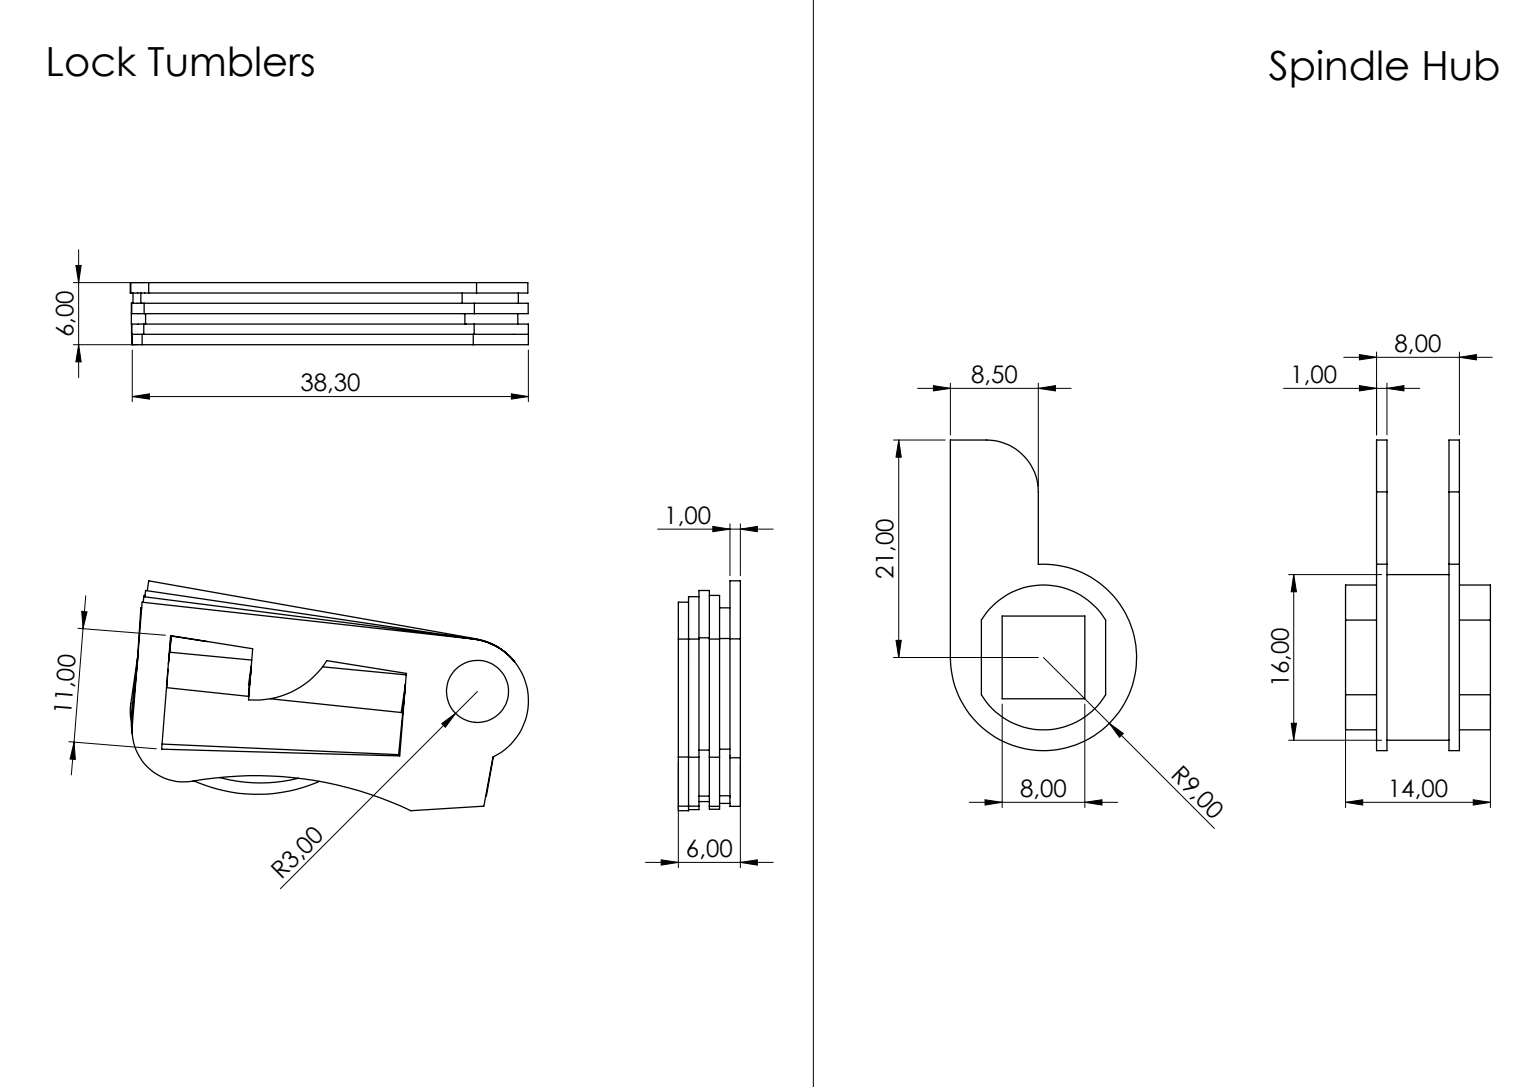
ISO-10303-21;
HEADER;
FILE_DESCRIPTION (('STEP AP214'),
    '1' );
FILE_NAME ('Spindle Hub.step',
    '2026-10-06T13:23:30',
    ( '' ),
    ( '' ),
    'SwSTEP 2.0',
    'SolidWorks 2020',
    '' );
FILE_SCHEMA (( 'AUTOMOTIVE_DESIGN' ));
ENDSEC;

DATA;
#2=FACE_OUTER_BOUND ( 'NONE', #19323, .T. ) ;
#35=FACE_OUTER_BOUND ( 'NONE', #21489, .T. ) ;
#39=ORIENTED_EDGE ( 'NONE', *, *, #18140, .F. ) ;
#55=ORIENTED_EDGE ( 'NONE', *, *, #18140, .T. ) ;
#134=LINE ( 'NONE', #14635, #4183 ) ;
#182=UNCERTAINTY_MEASURE_WITH_UNIT (LENGTH_MEASURE( 1.000000000000000082E-05 ), #19737, 'distance_accuracy_value', 'NONE');
#193=ORIENTED_EDGE ( 'NONE', *, *, #5602, .T. ) ;
#231=EDGE_CURVE ( 'NONE', #11233, #3677, #3985, .T. ) ;
#251=CARTESIAN_POINT ( 'NONE',  ( 10.50000000010000001, 20.50000000000000000, -150.5552959529999839 ) ) ;
#291=CARTESIAN_POINT ( 'NONE',  ( -0.7499999998410000757, 41.50000000000000000, -139.5552959529999839 ) ) ;
#295=ORIENTED_EDGE ( 'NONE', *, *, #21236, .T. ) ;
#312=DIRECTION ( 'NONE',  ( 2.257144641399999941E-12, -4.009147065140000298E-51, 1.000000000000000000 ) ) ;
#362=AXIS2_PLACEMENT_3D ( 'NONE', #6405, #22711, #20943 ) ;
#418=PLANE ( 'NONE',  #1885 ) ;
#426=FACE_OUTER_BOUND ( 'NONE', #14985, .T. ) ;
#436=ORIENTED_EDGE ( 'NONE', *, *, #7654, .T. ) ;
#439=ORIENTED_EDGE ( 'NONE', *, *, #4229, .F. ) ;
#486=AXIS2_PLACEMENT_3D ( 'NONE', #13907, #11751, #12111 ) ;
#542=ORIENTED_EDGE ( 'NONE', *, *, #17707, .F. ) ;
#547=DIRECTION ( 'NONE',  ( -2.257144641399999941E-12, 0.000000000000000000, -1.000000000000000000 ) ) ;
#628=CARTESIAN_POINT ( 'NONE',  ( 12.50000000010000001, 24.10555127549999810, -150.5552959529999839 ) ) ;
#665=ADVANCED_FACE ( 'NONE', ( #6439 ), #20974, .T. ) ;
#705=ORIENTED_EDGE ( 'NONE', *, *, #23377, .F. ) ;
#708=ORIENTED_EDGE ( 'NONE', *, *, #12053, .T. ) ;
#731=AXIS2_PLACEMENT_3D ( 'NONE', #8142, #11836, #22803 ) ;
#762=CARTESIAN_POINT ( 'NONE',  ( 12.50000000010000001, 20.50000000000000000, -147.5552959529999839 ) ) ;
#781=PRODUCT_DEFINITION ( 'UNKNOWN', '', #11904, #8501 ) ;
#813=CARTESIAN_POINT ( 'NONE',  ( 6.500000000149999124, 20.50000000000000000, -143.5552959529999839 ) ) ;
#855=ORIENTED_EDGE ( 'NONE', *, *, #15175, .F. ) ;
#860=ORIENTED_EDGE ( 'NONE', *, *, #19332, .F. ) ;
#899=FACE_OUTER_BOUND ( 'NONE', #6411, .T. ) ;
#901=CARTESIAN_POINT ( 'NONE',  ( 0.5000000001500000124, 16.89444872450000190, -143.5552959529999839 ) ) ;
#999=DIRECTION ( 'NONE',  ( 1.000000000000000000, 0.000000000000000000, -2.256131789327549967E-12 ) ) ;
#1028=CARTESIAN_POINT ( 'NONE',  ( 6.500000000159999125, 12.50000000000000000, -140.5552959529999839 ) ) ;
#1080=DIRECTION ( 'NONE',  ( 1.000000000000000000, -1.190078432789999897E-50, -2.257144641399999941E-12 ) ) ;
#1107=EDGE_CURVE ( 'NONE', #9556, #20751, #13681, .T. ) ;
#1109=EDGE_LOOP ( 'NONE', ( #4239, #8656, #12056, #15119 ) ) ;
#1120=DIRECTION ( 'NONE',  ( 2.257144641399999941E-12, -4.009147065140000298E-51, 1.000000000000000000 ) ) ;
#1121=VECTOR ( 'NONE', #19395, 1000.000000000000000 ) ;
#1130=ORIENTED_EDGE ( 'NONE', *, *, #23377, .T. ) ;
#1161=DIRECTION ( 'NONE',  ( 1.000000000000000000, 0.000000000000000000, 0.000000000000000000 ) ) ;
#1163=DIRECTION ( 'NONE',  ( 2.257144641399999941E-12, -4.009147065140000298E-51, 1.000000000000000000 ) ) ;
#1177=DIRECTION ( 'NONE',  ( 1.000000000000000000, 0.000000000000000000, -2.257453483404484831E-12 ) ) ;
#1188=DIRECTION ( 'NONE',  ( 1.000000000000000000, 0.000000000000000000, -2.257144641399999941E-12 ) ) ;
#1201=ORIENTED_EDGE ( 'NONE', *, *, #14324, .T. ) ;
#1232=ORIENTED_EDGE ( 'NONE', *, *, #20162, .F. ) ;
#1337=CARTESIAN_POINT ( 'NONE',  ( 1.000000000140000012, 41.50000000000000000, -147.0552959529999839 ) ) ;
#1349=CARTESIAN_POINT ( 'NONE',  ( 6.500000000140000012, 20.50000000000000000, -147.5552959529999839 ) ) ;
#1366=CARTESIAN_POINT ( 'NONE',  ( 2.500000000150000012, 24.50000000000000000, -143.5552959529999839 ) ) ;
#1369=VERTEX_POINT ( 'NONE', #15757 ) ;
#1379=EDGE_CURVE ( 'NONE', #9692, #10188, #2914, .T. ) ;
#1491=ORIENTED_EDGE ( 'NONE', *, *, #21184, .T. ) ;
#1565=CARTESIAN_POINT ( 'NONE',  ( -2.499999999859999988, 20.50000000000000000, -147.5552959529999839 ) ) ;
#1588=EDGE_CURVE ( 'NONE', #2933, #20660, #20036, .T. ) ;
#1620=CARTESIAN_POINT ( 'NONE',  ( 0.5000000001590000354, 20.50000000000000000, -139.5552959529999839 ) ) ;
#1692=ADVANCED_FACE ( 'NONE', ( #6899 ), #14167, .F. ) ;
#1695=EDGE_CURVE ( 'NONE', #8517, #8429, #19003, .T. ) ;
#1735=DIRECTION ( 'NONE',  ( 2.256861364460000137E-12, 0.000000000000000000, 1.000000000000000000 ) ) ;
#1788=CARTESIAN_POINT ( 'NONE',  ( -2.499999999839999987, 41.50000000000000000, -140.0552959529999839 ) ) ;
#1885=AXIS2_PLACEMENT_3D ( 'NONE', #17176, #2446, #9900 ) ;
#1915=CARTESIAN_POINT ( 'NONE',  ( -2.499999999839999987, 31.00000000000000000, -139.5552959529999839 ) ) ;
#1925=DIRECTION ( 'NONE',  ( 1.000000000000000000, 0.000000000000000000, -2.258609965721802837E-12 ) ) ;
#1960=CARTESIAN_POINT ( 'NONE',  ( -2.499999999859999988, 41.50000000000000000, -147.5552959529999839 ) ) ;
#2005=ORIENTED_EDGE ( 'NONE', *, *, #2166, .T. ) ;
#2013=ADVANCED_FACE ( 'NONE', ( #19771, #23333 ), #3696, .T. ) ;
#2034=DIRECTION ( 'NONE',  ( 1.000000000000000000, 0.000000000000000000, -2.257144641399999941E-12 ) ) ;
#2135=VECTOR ( 'NONE', #11700, 1000.000000000000000 ) ;
#2162=DIRECTION ( 'NONE',  ( 0.000000000000000000, -1.000000000000000000, 0.000000000000000000 ) ) ;
#2164=VERTEX_POINT ( 'NONE', #16015 ) ;
#2166=EDGE_CURVE ( 'NONE', #14118, #10634, #8177, .T. ) ;
#2167=AXIS2_PLACEMENT_3D ( 'NONE', #6419, #4646, #10091 ) ;
#2168=EDGE_LOOP ( 'NONE', ( #4075, #9774, #2218, #5035 ) ) ;
#2216=VECTOR ( 'NONE', #13785, 1000.000000000000000 ) ;
#2218=ORIENTED_EDGE ( 'NONE', *, *, #14621, .F. ) ;
#2254=ORIENTED_EDGE ( 'NONE', *, *, #12139, .F. ) ;
#2278=AXIS2_PLACEMENT_3D ( 'NONE', #12325, #19839, #14245 ) ;
#2285=DIRECTION ( 'NONE',  ( 1.000000000000000000, -1.190078432789999897E-50, -2.257144641399999941E-12 ) ) ;
#2341=ORIENTED_EDGE ( 'NONE', *, *, #15619, .F. ) ;
#2425=STYLED_ITEM ( 'NONE', ( #4984 ), #18345 ) ;
#2446=DIRECTION ( 'NONE',  ( 2.257144641399999941E-12, -4.009147065140000298E-51, 1.000000000000000000 ) ) ;
#2493=LINE ( 'NONE', #13417, #5918 ) ;
#2504=EDGE_LOOP ( 'NONE', ( #2554, #7882, #8397, #3230 ) ) ;
#2510=EDGE_LOOP ( 'NONE', ( #11261, #16222, #18656, #11978 ) ) ;
#2515=EDGE_CURVE ( 'NONE', #12071, #8946, #22656, .T. ) ;
#2531=DIRECTION ( 'NONE',  ( 2.257144641404620116E-12, 2.777754792983395132E-24, 1.000000000000000000 ) ) ;
#2538=DIRECTION ( 'NONE',  ( 0.000000000000000000, -1.000000000000000000, 0.000000000000000000 ) ) ;
#2540=ADVANCED_FACE ( 'NONE', ( #899 ), #4099, .F. ) ;
#2554=ORIENTED_EDGE ( 'NONE', *, *, #15296, .F. ) ;
#2632=DIRECTION ( 'NONE',  ( -2.257144641399999941E-12, 4.009147065140000298E-51, -1.000000000000000000 ) ) ;
#2653=APPLICATION_CONTEXT ( 'automotive_design' ) ;
#2665=CARTESIAN_POINT ( 'NONE',  ( 6.500000000170000014, 20.50000000000000000, -136.5552959530000123 ) ) ;
#2682=DIRECTION ( 'NONE',  ( 1.000000000000000000, -1.190078432789999897E-50, -2.257144641399999941E-12 ) ) ;
#2703=ORIENTED_EDGE ( 'NONE', *, *, #14053, .F. ) ;
#2716=VERTEX_POINT ( 'NONE', #23128 ) ;
#2740=FACE_OUTER_BOUND ( 'NONE', #2504, .T. ) ;
#2744=AXIS2_PLACEMENT_3D ( 'NONE', #22872, #2531, #4664 ) ;
#2748=DIRECTION ( 'NONE',  ( -2.257144641399999941E-12, 0.000000000000000000, -1.000000000000000000 ) ) ;
#2758=VERTEX_POINT ( 'NONE', #1960 ) ;
#2824=LINE ( 'NONE', #22941, #17455 ) ;
#2858=ORIENTED_EDGE ( 'NONE', *, *, #5935, .T. ) ;
#2869=DIRECTION ( 'NONE',  ( 3.882490197650000213E-51, -1.000000000000000000, -4.009147065150000317E-51 ) ) ;
#2874=AXIS2_PLACEMENT_3D ( 'NONE', #16722, #23523, #18291 ) ;
#2914=LINE ( 'NONE', #1366, #9859 ) ;
#2933=VERTEX_POINT ( 'NONE', #628 ) ;
#2954=ORIENTED_EDGE ( 'NONE', *, *, #12303, .T. ) ;
#3018=CARTESIAN_POINT ( 'NONE',  ( 2.500000000170000014, 24.50000000000000000, -136.5552959530000123 ) ) ;
#3046=DIRECTION ( 'NONE',  ( 0.000000000000000000, 1.000000000000000000, 0.000000000000000000 ) ) ;
#3063=ORIENTED_EDGE ( 'NONE', *, *, #19396, .T. ) ;
#3075=VERTEX_POINT ( 'NONE', #16916 ) ;
#3089=ORIENTED_EDGE ( 'NONE', *, *, #3888, .T. ) ;
#3121=CARTESIAN_POINT ( 'NONE',  ( 12.50000000020000002, 24.10555127549999810, -136.5552959530000123 ) ) ;
#3136=LINE ( 'NONE', #16093, #9380 ) ;
#3230=ORIENTED_EDGE ( 'NONE', *, *, #7654, .F. ) ;
#3281=DIRECTION ( 'NONE',  ( 1.000000000000000000, 0.000000000000000000, -2.256131789327550371E-12 ) ) ;
#3299=DIRECTION ( 'NONE',  ( 2.257115129720000004E-12, 0.000000000000000000, 1.000000000000000000 ) ) ;
#3387=VECTOR ( 'NONE', #12038, 1000.000000000000000 ) ;
#3463=DIRECTION ( 'NONE',  ( 2.257144641399999941E-12, -4.009147065140000298E-51, 1.000000000000000000 ) ) ;
#3481=VERTEX_POINT ( 'NONE', #18909 ) ;
#3519=VECTOR ( 'NONE', #15234, 1000.000000000000000 ) ;
#3567=DIRECTION ( 'NONE',  ( 3.882490197650000213E-51, -1.000000000000000000, -4.009147065150000317E-51 ) ) ;
#3607=ORIENTED_EDGE ( 'NONE', *, *, #10334, .T. ) ;
#3636=AXIS2_PLACEMENT_3D ( 'NONE', #5525, #11100, #23494 ) ;
#3648=DIRECTION ( 'NONE',  ( 2.257144641399999941E-12, 0.000000000000000000, 1.000000000000000000 ) ) ;
#3667=ORIENTED_EDGE ( 'NONE', *, *, #2515, .T. ) ;
#3677=VERTEX_POINT ( 'NONE', #17482 ) ;
#3678=CARTESIAN_POINT ( 'NONE',  ( 6.500000000140000012, 20.50000000000000000, -146.5552959529999839 ) ) ;
#3696=PLANE ( 'NONE',  #12169 ) ;
#3697=CARTESIAN_POINT ( 'NONE',  ( 6.500000000159999125, 20.50000000000000000, -139.5552959529999839 ) ) ;
#3745=CARTESIAN_POINT ( 'NONE',  ( 6.500000000140000012, 20.50000000000000000, -146.5552959529999839 ) ) ;
#3758=CARTESIAN_POINT ( 'NONE',  ( 6.500000000149999124, 12.50000000000000000, -143.5552959529999839 ) ) ;
#3762=CARTESIAN_POINT ( 'NONE',  ( 1.000000000160000013, 36.50000000000000000, -140.0552959529999839 ) ) ;
#3765=AXIS2_PLACEMENT_3D ( 'NONE', #11756, #1080, #2748 ) ;
#3857=VECTOR ( 'NONE', #3299, 1000.000000000000000 ) ;
#3881=VERTEX_POINT ( 'NONE', #5913 ) ;
#3888=EDGE_CURVE ( 'NONE', #8429, #10865, #16744, .T. ) ;
#3912=DIRECTION ( 'NONE',  ( 2.256988247090000272E-12, 0.000000000000000000, 1.000000000000000000 ) ) ;
#3961=LINE ( 'NONE', #1337, #23256 ) ;
#3980=ORIENTED_EDGE ( 'NONE', *, *, #17641, .F. ) ;
#3985=LINE ( 'NONE', #11218, #16794 ) ;
#4026=DIRECTION ( 'NONE',  ( 0.8571428571427679444, 0.5150787536378610421, -1.934960128632415569E-12 ) ) ;
#4075=ORIENTED_EDGE ( 'NONE', *, *, #23457, .F. ) ;
#4099=PLANE ( 'NONE',  #17649 ) ;
#4109=ADVANCED_FACE ( 'NONE', ( #6618 ), #18878, .T. ) ;
#4137=VECTOR ( 'NONE', #14049, 1000.000000000000000 ) ;
#4149=ORIENTED_EDGE ( 'NONE', *, *, #1588, .T. ) ;
#4172=CARTESIAN_POINT ( 'NONE',  ( 12.50000000010000001, 16.89444872450000190, -143.5552959529999839 ) ) ;
#4183=VECTOR ( 'NONE', #21903, 1000.000000000000000 ) ;
#4224=EDGE_CURVE ( 'NONE', #14338, #2164, #14719, .T. ) ;
#4229=EDGE_CURVE ( 'NONE', #21917, #14118, #5306, .T. ) ;
#4230=ORIENTED_EDGE ( 'NONE', *, *, #15873, .T. ) ;
#4239=ORIENTED_EDGE ( 'NONE', *, *, #12303, .F. ) ;
#4242=VECTOR ( 'NONE', #22137, 1000.000000000000000 ) ;
#4259=CARTESIAN_POINT ( 'NONE',  ( 6.500000000140000012, 12.50000000000000000, -146.5552959529999839 ) ) ;
#4288=LINE ( 'NONE', #251, #3519 ) ;
#4306=DIRECTION ( 'NONE',  ( 1.000000000000000000, 0.000000000000000000, -2.257144641399999941E-12 ) ) ;
#4387=EDGE_LOOP ( 'NONE', ( #11899, #9813, #15038, #4737, #7332 ) ) ;
#4440=FACE_OUTER_BOUND ( 'NONE', #19109, .T. ) ;
#4463=LINE ( 'NONE', #15052, #2135 ) ;
#4550=LINE ( 'NONE', #13709, #20192 ) ;
#4565=AXIS2_PLACEMENT_3D ( 'NONE', #10450, #21431, #8551 ) ;
#4590=CARTESIAN_POINT ( 'NONE',  ( 0.000000000000000000, 0.000000000000000000, 0.000000000000000000 ) ) ;
#4602=LINE ( 'NONE', #11718, #15573 ) ;
#4620=LINE ( 'NONE', #17342, #2216 ) ;
#4622=ORIENTED_EDGE ( 'NONE', *, *, #15648, .F. ) ;
#4636=PLANE ( 'NONE',  #486 ) ;
#4646=DIRECTION ( 'NONE',  ( 2.257144641399999941E-12, -4.009147065140000298E-51, 1.000000000000000000 ) ) ;
#4664=DIRECTION ( 'NONE',  ( -0.8571428571427679444, -0.5150787536378610421, 1.934960128632415569E-12 ) ) ;
#4736=FACE_OUTER_BOUND ( 'NONE', #23383, .T. ) ;
#4737=ORIENTED_EDGE ( 'NONE', *, *, #19081, .T. ) ;
#4748=ORIENTED_EDGE ( 'NONE', *, *, #5602, .F. ) ;
#4753=AXIS2_PLACEMENT_3D ( 'NONE', #17014, #2632, #9862 ) ;
#4757=EDGE_CURVE ( 'NONE', #17568, #9722, #13324, .T. ) ;
#4795=DIRECTION ( 'NONE',  ( 2.257144641404620116E-12, 2.777754792983395132E-24, 1.000000000000000000 ) ) ;
#4810=EDGE_LOOP ( 'NONE', ( #19167, #14249, #3607, #21619 ) ) ;
#4819=DIRECTION ( 'NONE',  ( 0.000000000000000000, -1.000000000000000000, 0.000000000000000000 ) ) ;
#4872=AXIS2_PLACEMENT_3D ( 'NONE', #5169, #12870, #23150 ) ;
#4891=ADVANCED_FACE ( 'NONE', ( #21067 ), #12002, .T. ) ;
#4950=EDGE_CURVE ( 'NONE', #10763, #5071, #22748, .T. ) ;
#4964=VECTOR ( 'NONE', #8838, 1000.000000000000000 ) ;
#4974=CARTESIAN_POINT ( 'NONE',  ( 0.5000000001340000333, 24.10555127549999810, -150.5552959529999839 ) ) ;
#4984=PRESENTATION_STYLE_ASSIGNMENT (( #19966 ) ) ;
#5010=EDGE_CURVE ( 'NONE', #3075, #8221, #18193, .T. ) ;
#5025=AXIS2_PLACEMENT_3D ( 'NONE', #4590, #17084, #1161 ) ;
#5032=EDGE_CURVE ( 'NONE', #17345, #12862, #21419, .T. ) ;
#5035=ORIENTED_EDGE ( 'NONE', *, *, #13018, .F. ) ;
#5062=LINE ( 'NONE', #12306, #11250 ) ;
#5070=CARTESIAN_POINT ( 'NONE',  ( 6.500000000159999125, 20.50000000000000000, -139.5552959529999839 ) ) ;
#5071=VERTEX_POINT ( 'NONE', #4259 ) ;
#5111=CARTESIAN_POINT ( 'NONE',  ( 0.5000000001659999915, 16.89444872450000190, -136.5552959530000123 ) ) ;
#5169=CARTESIAN_POINT ( 'NONE',  ( 6.500000000140000012, 20.50000000000000000, -147.5552959529999839 ) ) ;
#5170=AXIS2_PLACEMENT_3D ( 'NONE', #1349, #1120, #15847 ) ;
#5179=ADVANCED_FACE ( 'NONE', ( #5917 ), #18423, .T. ) ;
#5210=CARTESIAN_POINT ( 'NONE',  ( -0.7499999998590000105, 41.50000000000000000, -147.5552959529999839 ) ) ;
#5222=DIRECTION ( 'NONE',  ( 0.000000000000000000, 4.009147065150000317E-51, -1.000000000000000000 ) ) ;
#5257=ORIENTED_EDGE ( 'NONE', *, *, #16090, .T. ) ;
#5282=FACE_OUTER_BOUND ( 'NONE', #2510, .T. ) ;
#5306=LINE ( 'NONE', #14239, #17777 ) ;
#5338=AXIS2_PLACEMENT_3D ( 'NONE', #901, #2682, #8371 ) ;
#5369=AXIS2_PLACEMENT_3D ( 'NONE', #6275, #13783, #17460 ) ;
#5474=EDGE_LOOP ( 'NONE', ( #21908, #2254, #20686, #10327, #9134 ) ) ;
#5496=CARTESIAN_POINT ( 'NONE',  ( 6.500000000149999124, 20.50000000000000000, -143.5552959529999839 ) ) ;
#5525=CARTESIAN_POINT ( 'NONE',  ( 1.000000000140000012, 36.50000000000000000, -147.5552959529999839 ) ) ;
#5548=CYLINDRICAL_SURFACE ( 'NONE', #2874, 7.000000000000000888 ) ;
#5579=FACE_BOUND ( 'NONE', #14822, .T. ) ;
#5584=CARTESIAN_POINT ( 'NONE',  ( 6.000000000140000012, 29.48610037779999971, -147.5552959529999839 ) ) ;
#5602=EDGE_CURVE ( 'NONE', #21645, #9539, #17282, .T. ) ;
#5649=VECTOR ( 'NONE', #2162, 1000.000000000000000 ) ;
#5694=FACE_OUTER_BOUND ( 'NONE', #5474, .T. ) ;
#5731=FACE_BOUND ( 'NONE', #2168, .T. ) ;
#5901=EDGE_LOOP ( 'NONE', ( #14706, #6579, #1130, #193 ) ) ;
#5913=CARTESIAN_POINT ( 'NONE',  ( 0.5000000001409999895, 24.10555127549999810, -147.5552959529999839 ) ) ;
#5917=FACE_OUTER_BOUND ( 'NONE', #10664, .T. ) ;
#5918=VECTOR ( 'NONE', #11272, 1000.000000000000000 ) ;
#5935=EDGE_CURVE ( 'NONE', #9692, #10310, #9707, .T. ) ;
#6042=CARTESIAN_POINT ( 'NONE',  ( 2.500000000170000014, 20.50000000000000000, -136.5552959530000123 ) ) ;
#6071=PLANE ( 'NONE',  #14780 ) ;
#6080=CIRCLE ( 'NONE', #22036, 8.000000000000000000 ) ;
#6088=CARTESIAN_POINT ( 'NONE',  ( 6.500000000130000011, 20.50000000000000000, -150.5552959529999839 ) ) ;
#6119=DIRECTION ( 'NONE',  ( 1.000000000000000000, -1.190078432789999897E-50, -2.257144641399999941E-12 ) ) ;
#6164=FACE_OUTER_BOUND ( 'NONE', #16658, .T. ) ;
#6165=EDGE_LOOP ( 'NONE', ( #14502, #11106, #20432, #855 ) ) ;
#6180=CARTESIAN_POINT ( 'NONE',  ( -2.499999999859999988, 31.00000000000000000, -146.5552959529999839 ) ) ;
#6218=( LENGTH_UNIT ( ) NAMED_UNIT ( * ) SI_UNIT ( .MILLI., .METRE. ) );
#6220=CARTESIAN_POINT ( 'NONE',  ( 10.50000000010000001, 24.50000000000000000, -143.5552959529999839 ) ) ;
#6221=ORIENTED_EDGE ( 'NONE', *, *, #10078, .T. ) ;
#6256=CARTESIAN_POINT ( 'NONE',  ( 6.500000000159999125, 20.50000000000000000, -140.5552959529999839 ) ) ;
#6260=ORIENTED_EDGE ( 'NONE', *, *, #14724, .T. ) ;
#6273=AXIS2_PLACEMENT_3D ( 'NONE', #813, #17211, #13772 ) ;
#6275=CARTESIAN_POINT ( 'NONE',  ( 6.500000000149999124, 20.50000000000000000, -143.5552959529999839 ) ) ;
#6328=SURFACE_STYLE_USAGE ( .BOTH. , #17036 ) ;
#6337=LINE ( 'NONE', #10011, #3387 ) ;
#6354=ORIENTED_EDGE ( 'NONE', *, *, #5010, .F. ) ;
#6358=VECTOR ( 'NONE', #7876, 1000.000000000000000 ) ;
#6370=PLANE ( 'NONE',  #731 ) ;
#6405=CARTESIAN_POINT ( 'NONE',  ( 6.500000000140000012, 20.50000000000000000, -147.0552959529999839 ) ) ;
#6411=EDGE_LOOP ( 'NONE', ( #6881, #708, #14928, #860 ) ) ;
#6413=CARTESIAN_POINT ( 'NONE',  ( 6.000000000160000013, 36.50000000000000000, -140.5552959529999839 ) ) ;
#6419=CARTESIAN_POINT ( 'NONE',  ( 6.500000000140000012, 20.50000000000000000, -147.5552959529999839 ) ) ;
#6437=CARTESIAN_POINT ( 'NONE',  ( 6.000000000140000012, 29.48610037779999971, -146.5552959529999839 ) ) ;
#6439=FACE_OUTER_BOUND ( 'NONE', #7445, .T. ) ;
#6450=VECTOR ( 'NONE', #12340, 1000.000000000000000 ) ;
#6474=EDGE_CURVE ( 'NONE', #17870, #8517, #16492, .T. ) ;
#6519=FACE_BOUND ( 'NONE', #6641, .T. ) ;
#6579=ORIENTED_EDGE ( 'NONE', *, *, #19941, .F. ) ;
#6618=FACE_OUTER_BOUND ( 'NONE', #4810, .T. ) ;
#6621=ORIENTED_EDGE ( 'NONE', *, *, #14621, .T. ) ;
#6641=EDGE_LOOP ( 'NONE', ( #542, #5257, #4230, #10402 ) ) ;
#6687=CARTESIAN_POINT ( 'NONE',  ( 1.000000000140000012, 41.50000000000000000, -147.5552959529999839 ) ) ;
#6709=DIRECTION ( 'NONE',  ( 1.000000000000000000, 0.000000000000000000, -2.258609965721802837E-12 ) ) ;
#6735=EDGE_CURVE ( 'NONE', #12862, #8946, #7107, .T. ) ;
#6813=ORIENTED_EDGE ( 'NONE', *, *, #1107, .T. ) ;
#6852=CARTESIAN_POINT ( 'NONE',  ( 1.000000000160000013, 36.50000000000000000, -139.5552959529999839 ) ) ;
#6881=ORIENTED_EDGE ( 'NONE', *, *, #16129, .F. ) ;
#6899=FACE_OUTER_BOUND ( 'NONE', #14811, .T. ) ;
#6918=ORIENTED_EDGE ( 'NONE', *, *, #2515, .F. ) ;
#6951=PLANE ( 'NONE',  #23169 ) ;
#6969=VERTEX_POINT ( 'NONE', #6687 ) ;
#6980=ORIENTED_EDGE ( 'NONE', *, *, #10262, .T. ) ;
#6985=EDGE_CURVE ( 'NONE', #1369, #21363, #3136, .T. ) ;
#7022=DIRECTION ( 'NONE',  ( -1.000000000000000000, 0.000000000000000000, 2.257495777610000006E-12 ) ) ;
#7023=CARTESIAN_POINT ( 'NONE',  ( 6.500000000140000012, 20.50000000000000000, -146.5552959529999839 ) ) ;
#7103=LINE ( 'NONE', #10534, #3857 ) ;
#7107=CIRCLE ( 'NONE', #14701, 7.000000000000000888 ) ;
#7141=CARTESIAN_POINT ( 'NONE',  ( 0.5000000001590284571, 24.10555127549999810, -139.5552959530157864 ) ) ;
#7159=DIRECTION ( 'NONE',  ( 2.257749542879999954E-12, 0.000000000000000000, 1.000000000000000000 ) ) ;
#7215=DIRECTION ( 'NONE',  ( 1.000000000000000000, 0.000000000000000000, -2.259303855112193156E-12 ) ) ;
#7272=AXIS2_PLACEMENT_3D ( 'NONE', #5070, #12313, #3281 ) ;
#7327=ADVANCED_FACE ( 'NONE', ( #5579, #5694 ), #18539, .F. ) ;
#7332=ORIENTED_EDGE ( 'NONE', *, *, #1107, .F. ) ;
#7350=MECHANICAL_DESIGN_GEOMETRIC_PRESENTATION_REPRESENTATION('',(#2425),#15705);
#7394=CARTESIAN_POINT ( 'NONE',  ( 1.000000000160000013, 41.50000000000000000, -140.0552959529999839 ) ) ;
#7441=CARTESIAN_POINT ( 'NONE',  ( 6.500000000130000011, 20.50000000000000000, -150.5552959529999839 ) ) ;
#7445=EDGE_LOOP ( 'NONE', ( #3089, #11834, #10733, #12920 ) ) ;
#7486=CARTESIAN_POINT ( 'NONE',  ( 6.000000000140000012, 29.48610037779999971, -147.0552959529999839 ) ) ;
#7559=AXIS2_PLACEMENT_3D ( 'NONE', #13641, #17449, #1177 ) ;
#7652=PLANE ( 'NONE',  #9752 ) ;
#7654=EDGE_CURVE ( 'NONE', #10634, #9455, #10931, .T. ) ;
#7669=ORIENTED_EDGE ( 'NONE', *, *, #14763, .F. ) ;
#7680=ORIENTED_EDGE ( 'NONE', *, *, #14053, .T. ) ;
#7730=DIRECTION ( 'NONE',  ( 0.000000000000000000, 1.000000000000000000, 0.000000000000000000 ) ) ;
#7739=CARTESIAN_POINT ( 'NONE',  ( 12.50000000020000002, 24.10555127549999810, -139.5552959529999839 ) ) ;
#7775=DIRECTION ( 'NONE',  ( 0.000000000000000000, 4.009147065150000317E-51, -1.000000000000000000 ) ) ;
#7835=CARTESIAN_POINT ( 'NONE',  ( -2.499999999839999987, 20.50000000000000000, -140.5552959529999839 ) ) ;
#7876=DIRECTION ( 'NONE',  ( -1.000000000000000000, 0.000000000000000000, 2.257495777610000006E-12 ) ) ;
#7882=ORIENTED_EDGE ( 'NONE', *, *, #20439, .T. ) ;
#7915=ORIENTED_EDGE ( 'NONE', *, *, #4757, .F. ) ;
#7927=CIRCLE ( 'NONE', #2278, 6.999999999999999112 ) ;
#7934=CYLINDRICAL_SURFACE ( 'NONE', #23221, 9.000000000000000000 ) ;
#7960=ORIENTED_EDGE ( 'NONE', *, *, #231, .T. ) ;
#7987=FILL_AREA_STYLE_COLOUR ( '', #18286 ) ;
#7996=LINE ( 'NONE', #291, #6358 ) ;
#7999=MECHANICAL_DESIGN_GEOMETRIC_PRESENTATION_REPRESENTATION('',(#22450),#17508);
#8076=FACE_OUTER_BOUND ( 'NONE', #23407, .T. ) ;
#8142=CARTESIAN_POINT ( 'NONE',  ( 2.500000000170000014, 16.50000000000000000, -136.5552959530000123 ) ) ;
#8176=( LENGTH_UNIT ( ) NAMED_UNIT ( * ) SI_UNIT ( .MILLI., .METRE. ) );
#8177=LINE ( 'NONE', #6180, #19016 ) ;
#8184=VECTOR ( 'NONE', #1735, 1000.000000000000000 ) ;
#8192=ORIENTED_EDGE ( 'NONE', *, *, #20666, .T. ) ;
#8221=VERTEX_POINT ( 'NONE', #9020 ) ;
#8286=ORIENTED_EDGE ( 'NONE', *, *, #18549, .F. ) ;
#8288=EDGE_CURVE ( 'NONE', #14413, #20358, #6080, .T. ) ;
#8326=VECTOR ( 'NONE', #8347, 1000.000000000000000 ) ;
#8331=EDGE_CURVE ( 'NONE', #11233, #17345, #134, .T. ) ;
#8332=DIRECTION ( 'NONE',  ( -1.000000000000000000, 0.000000000000000000, 2.255973186040000320E-12 ) ) ;
#8347=DIRECTION ( 'NONE',  ( 2.256861364460000137E-12, 0.000000000000000000, 1.000000000000000000 ) ) ;
#8367=DIRECTION ( 'NONE',  ( 2.256988247090000272E-12, 0.000000000000000000, 1.000000000000000000 ) ) ;
#8371=DIRECTION ( 'NONE',  ( -2.257144641399999941E-12, 0.000000000000000000, -1.000000000000000000 ) ) ;
#8397=ORIENTED_EDGE ( 'NONE', *, *, #12222, .T. ) ;
#8413=VECTOR ( 'NONE', #7022, 1000.000000000000000 ) ;
#8429=VERTEX_POINT ( 'NONE', #20459 ) ;
#8442=CARTESIAN_POINT ( 'NONE',  ( 10.50000000020000002, 24.50000000000000000, -136.5552959530000123 ) ) ;
#8481=ORIENTED_EDGE ( 'NONE', *, *, #15619, .T. ) ;
#8501=PRODUCT_DEFINITION_CONTEXT ( 'detailed design', #22556, 'design' ) ;
#8517=VERTEX_POINT ( 'NONE', #17593 ) ;
#8551=DIRECTION ( 'NONE',  ( 1.000000000000000000, 0.000000000000000000, -2.256131789327550371E-12 ) ) ;
#8647=CARTESIAN_POINT ( 'NONE',  ( 0.5000000001500000124, 16.89444872450000190, -143.5552959529999839 ) ) ;
#8655=ADVANCED_FACE ( 'NONE', ( #5282 ), #6951, .F. ) ;
#8656=ORIENTED_EDGE ( 'NONE', *, *, #8331, .F. ) ;
#8657=PLANE ( 'NONE',  #20399 ) ;
#8700=VECTOR ( 'NONE', #11915, 1000.000000000000000 ) ;
#8716=EDGE_CURVE ( 'NONE', #3075, #9674, #18021, .T. ) ;
#8718=CARTESIAN_POINT ( 'NONE',  ( 0.5000000001409999895, 16.89444872450000190, -147.5552959529999839 ) ) ;
#8720=CARTESIAN_POINT ( 'NONE',  ( -2.499999999839999987, 31.00000000000000000, -140.5552959529999839 ) ) ;
#8838=DIRECTION ( 'NONE',  ( 0.000000000000000000, -1.000000000000000000, 0.000000000000000000 ) ) ;
#8895=DIRECTION ( 'NONE',  ( 2.257144641399999941E-12, -4.009147065140000298E-51, 1.000000000000000000 ) ) ;
#8946=VERTEX_POINT ( 'NONE', #12697 ) ;
#8964=EDGE_LOOP ( 'NONE', ( #4149, #14685, #19803, #8192 ) ) ;
#8965=CIRCLE ( 'NONE', #2167, 7.000000000000000888 ) ;
#8984=DIRECTION ( 'NONE',  ( 1.000000000000000000, 0.000000000000000000, -2.256131789327550371E-12 ) ) ;
#8998=ORIENTED_EDGE ( 'NONE', *, *, #16843, .F. ) ;
#9002=DIRECTION ( 'NONE',  ( 1.000000000000000000, -1.190078432789999897E-50, -2.257144641399999941E-12 ) ) ;
#9020=CARTESIAN_POINT ( 'NONE',  ( -2.499999999839999987, 41.50000000000000000, -139.5552959529999839 ) ) ;
#9030=ORIENTED_EDGE ( 'NONE', *, *, #12726, .F. ) ;
#9078=ADVANCED_FACE ( 'NONE', ( #13160 ), #20429, .T. ) ;
#9119=SHAPE_REPRESENTATION_RELATIONSHIP ( 'NONE' , 'NONE' ,  #17559, #18345 ) ;
#9134=ORIENTED_EDGE ( 'NONE', *, *, #12053, .F. ) ;
#9152=PLANE ( 'NONE',  #19343 ) ;
#9210=ORIENTED_EDGE ( 'NONE', *, *, #16129, .T. ) ;
#9229=ORIENTED_EDGE ( 'NONE', *, *, #2166, .F. ) ;
#9293=ORIENTED_EDGE ( 'NONE', *, *, #12139, .T. ) ;
#9347=CIRCLE ( 'NONE', #15822, 8.000000000000000000 ) ;
#9355=CARTESIAN_POINT ( 'NONE',  ( 6.500000000149999124, 20.50000000000000000, -143.5552959529999839 ) ) ;
#9380=VECTOR ( 'NONE', #7159, 1000.000000000000000 ) ;
#9389=ORIENTED_EDGE ( 'NONE', *, *, #18564, .T. ) ;
#9397=AXIS2_PLACEMENT_3D ( 'NONE', #3745, #9422, #16699 ) ;
#9422=DIRECTION ( 'NONE',  ( 2.257144641399999941E-12, -4.009147065140000298E-51, 1.000000000000000000 ) ) ;
#9442=VECTOR ( 'NONE', #15211, 1000.000000000000000 ) ;
#9455=VERTEX_POINT ( 'NONE', #6437 ) ;
#9471=CARTESIAN_POINT ( 'NONE',  ( 10.50000000020000002, 16.50000000000000000, -136.5552959530000123 ) ) ;
#9498=LINE ( 'NONE', #7486, #4242 ) ;
#9501=CARTESIAN_POINT ( 'NONE',  ( 6.000000000140000012, 36.50000000000000000, -147.5552959529999839 ) ) ;
#9539=VERTEX_POINT ( 'NONE', #19415 ) ;
#9556=VERTEX_POINT ( 'NONE', #12258 ) ;
#9649=ADVANCED_FACE ( 'NONE', ( #12616, #23334 ), #9152, .T. ) ;
#9674=VERTEX_POINT ( 'NONE', #7835 ) ;
#9692=VERTEX_POINT ( 'NONE', #13544 ) ;
#9707=LINE ( 'NONE', #6042, #9442 ) ;
#9722=VERTEX_POINT ( 'NONE', #9501 ) ;
#9752=AXIS2_PLACEMENT_3D ( 'NONE', #14923, #22180, #11562 ) ;
#9774=ORIENTED_EDGE ( 'NONE', *, *, #11692, .F. ) ;
#9775=FACE_BOUND ( 'NONE', #13425, .T. ) ;
#9795=VERTEX_POINT ( 'NONE', #13195 ) ;
#9809=EDGE_LOOP ( 'NONE', ( #6260, #22002, #17630, #9293 ) ) ;
#9813=ORIENTED_EDGE ( 'NONE', *, *, #16514, .T. ) ;
#9819=AXIS2_PLACEMENT_3D ( 'NONE', #3678, #8895, #21537 ) ;
#9859=VECTOR ( 'NONE', #14092, 1000.000000000000000 ) ;
#9862=DIRECTION ( 'NONE',  ( 1.000000000000000000, 0.000000000000000000, -2.259303855112193560E-12 ) ) ;
#9874=ADVANCED_FACE ( 'NONE', ( #2740 ), #12109, .T. ) ;
#9888=ORIENTED_EDGE ( 'NONE', *, *, #6735, .T. ) ;
#9900=DIRECTION ( 'NONE',  ( 1.000000000000000000, 0.000000000000000000, -2.257144641399999941E-12 ) ) ;
#9957=ORIENTED_EDGE ( 'NONE', *, *, #17641, .T. ) ;
#9976=PRODUCT_DEFINITION_SHAPE ( 'NONE', 'NONE',  #781 ) ;
#10002=EDGE_LOOP ( 'NONE', ( #22288, #12519, #2858, #22933 ) ) ;
#10011=CARTESIAN_POINT ( 'NONE',  ( 6.500000000149999124, 28.50000000000000000, -143.5552959529999839 ) ) ;
#10078=EDGE_CURVE ( 'NONE', #6969, #2758, #23420, .T. ) ;
#10091=DIRECTION ( 'NONE',  ( 1.000000000000000000, 0.000000000000000000, -2.256131789327549967E-12 ) ) ;
#10103=DIRECTION ( 'NONE',  ( 0.000000000000000000, 4.009147065150000317E-51, -1.000000000000000000 ) ) ;
#10188=VERTEX_POINT ( 'NONE', #21029 ) ;
#10190=DIRECTION ( 'NONE',  ( 2.257144641399999941E-12, -4.009147065140000298E-51, 1.000000000000000000 ) ) ;
#10204=AXIS2_PLACEMENT_3D ( 'NONE', #15417, #1163, #18992 ) ;
#10210=VECTOR ( 'NONE', #13550, 1000.000000000000000 ) ;
#10215=CARTESIAN_POINT ( 'NONE',  ( 0.5000000001500000124, 16.89444872450000190, -143.5552959529999839 ) ) ;
#10262=EDGE_CURVE ( 'NONE', #9795, #21893, #4602, .T. ) ;
#10310=VERTEX_POINT ( 'NONE', #18041 ) ;
#10319=DIRECTION ( 'NONE',  ( 0.000000000000000000, 1.000000000000000000, 0.000000000000000000 ) ) ;
#10327=ORIENTED_EDGE ( 'NONE', *, *, #8716, .F. ) ;
#10328=VECTOR ( 'NONE', #10319, 1000.000000000000000 ) ;
#10334=EDGE_CURVE ( 'NONE', #5071, #20358, #15892, .T. ) ;
#10399=UNCERTAINTY_MEASURE_WITH_UNIT (LENGTH_MEASURE( 1.000000000000000082E-05 ), #6218, 'distance_accuracy_value', 'NONE');
#10402=ORIENTED_EDGE ( 'NONE', *, *, #18549, .T. ) ;
#10450=CARTESIAN_POINT ( 'NONE',  ( 6.500000000130000011, 20.50000000000000000, -150.5552959529999839 ) ) ;
#10475=PLANE ( 'NONE',  #13147 ) ;
#10527=ADVANCED_FACE ( 'NONE', ( #12906 ), #20187, .F. ) ;
#10534=CARTESIAN_POINT ( 'NONE',  ( 0.5000000001500000124, 24.10555127549999810, -143.5552959529999839 ) ) ;
#10544=ADVANCED_FACE ( 'NONE', ( #426 ), #21002, .F. ) ;
#10547=FILL_AREA_STYLE ('',( #18181 ) ) ;
#10566=AXIS2_PLACEMENT_3D ( 'NONE', #9355, #16626, #4026 ) ;
#10570=CARTESIAN_POINT ( 'NONE',  ( 6.000000000160000013, 36.50000000000000000, -139.5552959529999839 ) ) ;
#10584=ORIENTED_EDGE ( 'NONE', *, *, #5032, .F. ) ;
#10617=LINE ( 'NONE', #1620, #4964 ) ;
#10634=VERTEX_POINT ( 'NONE', #13965 ) ;
#10648=CYLINDRICAL_SURFACE ( 'NONE', #14083, 5.000000000000000888 ) ;
#10664=EDGE_LOOP ( 'NONE', ( #2954, #3667, #21768, #10584 ) ) ;
#10733=ORIENTED_EDGE ( 'NONE', *, *, #18564, .F. ) ;
#10740=DIRECTION ( 'NONE',  ( 1.000000000000000000, -1.190078432789999897E-50, -2.257144641399999941E-12 ) ) ;
#10763=VERTEX_POINT ( 'NONE', #23368 ) ;
#10786=ORIENTED_EDGE ( 'NONE', *, *, #10334, .F. ) ;
#10865=VERTEX_POINT ( 'NONE', #22875 ) ;
#10931=CIRCLE ( 'NONE', #9397, 9.000000000000000000 ) ;
#10932=DIRECTION ( 'NONE',  ( 1.000000000000000000, 0.000000000000000000, -2.257144641399999941E-12 ) ) ;
#10947=VECTOR ( 'NONE', #3912, 1000.000000000000000 ) ;
#11005=FACE_OUTER_BOUND ( 'NONE', #18107, .T. ) ;
#11028=VECTOR ( 'NONE', #2538, 1000.000000000000000 ) ;
#11036=CARTESIAN_POINT ( 'NONE',  ( 6.500000000159999125, 28.50000000000000000, -140.5552959529999839 ) ) ;
#11065=ORIENTED_EDGE ( 'NONE', *, *, #11527, .T. ) ;
#11100=DIRECTION ( 'NONE',  ( 2.257144641399999941E-12, -4.009147065140000298E-51, 1.000000000000000000 ) ) ;
#11106=ORIENTED_EDGE ( 'NONE', *, *, #1695, .F. ) ;
#11176=CARTESIAN_POINT ( 'NONE',  ( -2.499999999859999988, 41.50000000000000000, -146.5552959529999839 ) ) ;
#11216=AXIS2_PLACEMENT_3D ( 'NONE', #19244, #10190, #1188 ) ;
#11218=CARTESIAN_POINT ( 'NONE',  ( 12.50000000010000001, 16.89444872450000190, -143.5552959529999839 ) ) ;
#11223=ADVANCED_FACE ( 'NONE', ( #11005 ), #10648, .T. ) ;
#11233=VERTEX_POINT ( 'NONE', #12679 ) ;
#11240=VERTEX_POINT ( 'NONE', #14241 ) ;
#11250=VECTOR ( 'NONE', #19578, 1000.000000000000000 ) ;
#11261=ORIENTED_EDGE ( 'NONE', *, *, #15648, .T. ) ;
#11272=DIRECTION ( 'NONE',  ( 0.000000000000000000, 1.000000000000000000, 0.000000000000000000 ) ) ;
#11288=AXIS2_PLACEMENT_3D ( 'NONE', #15740, #14076, #21106 ) ;
#11493=EDGE_LOOP ( 'NONE', ( #6918, #11065, #6980, #2703 ) ) ;
#11527=EDGE_CURVE ( 'NONE', #12071, #9795, #10617, .T. ) ;
#11548=EDGE_CURVE ( 'NONE', #2758, #18780, #22172, .T. ) ;
#11562=DIRECTION ( 'NONE',  ( -2.257144641399999941E-12, 0.000000000000000000, -1.000000000000000000 ) ) ;
#11692=EDGE_CURVE ( 'NONE', #11694, #10188, #4550, .T. ) ;
#11693=MANIFOLD_SOLID_BREP ( 'Stock-MAS-159-1', #13340 ) ;
#11694=VERTEX_POINT ( 'NONE', #11790 ) ;
#11700=DIRECTION ( 'NONE',  ( 2.257749542879999954E-12, 0.000000000000000000, 1.000000000000000000 ) ) ;
#11713=DIRECTION ( 'NONE',  ( 1.000000000000000000, 0.000000000000000000, -2.257453483404484831E-12 ) ) ;
#11718=CARTESIAN_POINT ( 'NONE',  ( 0.5000000001500000124, 16.89444872450000190, -143.5552959529999839 ) ) ;
#11751=DIRECTION ( 'NONE',  ( -1.000000000000000000, 1.190078432789999897E-50, 2.257144641399999941E-12 ) ) ;
#11756=CARTESIAN_POINT ( 'NONE',  ( 12.50000000010000001, 16.89444872450000190, -143.5552959529999839 ) ) ;
#11790=CARTESIAN_POINT ( 'NONE',  ( 2.500000000130000011, 16.50000000000000000, -150.5552959529999839 ) ) ;
#11834=ORIENTED_EDGE ( 'NONE', *, *, #16090, .F. ) ;
#11836=DIRECTION ( 'NONE',  ( -1.000000000000000000, 1.190078432789999897E-50, 2.257144641399999941E-12 ) ) ;
#11899=ORIENTED_EDGE ( 'NONE', *, *, #19332, .T. ) ;
#11904=PRODUCT_DEFINITION_FORMATION_WITH_SPECIFIED_SOURCE ( 'ANY', '', #21028, .NOT_KNOWN. ) ;
#11915=DIRECTION ( 'NONE',  ( -2.257115129720000004E-12, 0.000000000000000000, -1.000000000000000000 ) ) ;
#11978=ORIENTED_EDGE ( 'NONE', *, *, #4757, .T. ) ;
#11980=PLANE ( 'NONE',  #11216 ) ;
#12002=PLANE ( 'NONE',  #3765 ) ;
#12038=DIRECTION ( 'NONE',  ( 2.257157423930000049E-12, 0.000000000000000000, 1.000000000000000000 ) ) ;
#12042=VECTOR ( 'NONE', #13039, 1000.000000000000000 ) ;
#12053=EDGE_CURVE ( 'NONE', #2164, #3075, #12486, .T. ) ;
#12056=ORIENTED_EDGE ( 'NONE', *, *, #15044, .F. ) ;
#12063=CARTESIAN_POINT ( 'NONE',  ( 12.50000000020000002, 20.50000000000000000, -136.5552959530000123 ) ) ;
#12071=VERTEX_POINT ( 'NONE', #7141 ) ;
#12073=CIRCLE ( 'NONE', #4872, 9.000000000000000000 ) ;
#12102=CARTESIAN_POINT ( 'NONE',  ( 10.50000000020000002, 20.50000000000000000, -136.5552959530000123 ) ) ;
#12109=CYLINDRICAL_SURFACE ( 'NONE', #362, 9.000000000000000000 ) ;
#12111=DIRECTION ( 'NONE',  ( 1.190078432789999897E-50, 1.000000000000000000, 0.000000000000000000 ) ) ;
#12139=EDGE_CURVE ( 'NONE', #1369, #14338, #14404, .T. ) ;
#12158=DIRECTION ( 'NONE',  ( 0.000000000000000000, 4.009147065150000317E-51, -1.000000000000000000 ) ) ;
#12169=AXIS2_PLACEMENT_3D ( 'NONE', #7023, #3463, #10932 ) ;
#12222=EDGE_CURVE ( 'NONE', #17568, #9455, #9498, .T. ) ;
#12230=ORIENTED_EDGE ( 'NONE', *, *, #22174, .F. ) ;
#12258=CARTESIAN_POINT ( 'NONE',  ( 1.000000000160000013, 41.50000000000000000, -139.5552959529999839 ) ) ;
#12260=LINE ( 'NONE', #17387, #16796 ) ;
#12268=CARTESIAN_POINT ( 'NONE',  ( 6.500000000170000014, 16.50000000000000000, -136.5552959530000123 ) ) ;
#12303=EDGE_CURVE ( 'NONE', #17345, #12071, #17529, .T. ) ;
#12306=CARTESIAN_POINT ( 'NONE',  ( 6.000000000160000013, 32.99305018889999275, -139.5552959529999839 ) ) ;
#12313=DIRECTION ( 'NONE',  ( 2.257144641399999941E-12, -4.009147065140000298E-51, 1.000000000000000000 ) ) ;
#12320=DIRECTION ( 'NONE',  ( -1.000000000000000000, 0.000000000000000000, 2.257495777610000006E-12 ) ) ;
#12325=CARTESIAN_POINT ( 'NONE',  ( 6.500000000159999125, 20.50000000000000000, -139.5552959529999839 ) ) ;
#12335=EDGE_LOOP ( 'NONE', ( #3980, #14157, #22062, #9229 ) ) ;
#12340=DIRECTION ( 'NONE',  ( -1.000000000000000000, 0.000000000000000000, 2.257495777610000006E-12 ) ) ;
#12364=VECTOR ( 'NONE', #3046, 1000.000000000000000 ) ;
#12458=( NAMED_UNIT ( * ) PLANE_ANGLE_UNIT ( ) SI_UNIT ( $, .RADIAN. ) );
#12478=VECTOR ( 'NONE', #21888, 1000.000000000000000 ) ;
#12486=LINE ( 'NONE', #21553, #8413 ) ;
#12508=ORIENTED_EDGE ( 'NONE', *, *, #12736, .T. ) ;
#12519=ORIENTED_EDGE ( 'NONE', *, *, #1379, .F. ) ;
#12542=UNCERTAINTY_MEASURE_WITH_UNIT (LENGTH_MEASURE( 1.000000000000000082E-05 ), #8176, 'distance_accuracy_value', 'NONE');
#12543=ORIENTED_EDGE ( 'NONE', *, *, #6474, .T. ) ;
#12592=CARTESIAN_POINT ( 'NONE',  ( 12.50000000010000001, 24.10555127549999810, -143.5552959529999839 ) ) ;
#12616=FACE_BOUND ( 'NONE', #1109, .T. ) ;
#12628=AXIS2_PLACEMENT_3D ( 'NONE', #8647, #9002, #12702 ) ;
#12679=CARTESIAN_POINT ( 'NONE',  ( 12.50000000010902745, 16.89444872450000190, -139.5552959530157864 ) ) ;
#12697=CARTESIAN_POINT ( 'NONE',  ( 0.5000000001659999915, 24.10555127549999810, -136.5552959530000123 ) ) ;
#12702=DIRECTION ( 'NONE',  ( -2.257144641399999941E-12, 0.000000000000000000, -1.000000000000000000 ) ) ;
#12726=EDGE_CURVE ( 'NONE', #6969, #21917, #3961, .T. ) ;
#12736=EDGE_CURVE ( 'NONE', #21645, #9692, #12260, .T. ) ;
#12862=VERTEX_POINT ( 'NONE', #3121 ) ;
#12867=DIRECTION ( 'NONE',  ( 2.257144641399999941E-12, -4.009147065140000298E-51, 1.000000000000000000 ) ) ;
#12870=DIRECTION ( 'NONE',  ( 2.257144641399999941E-12, -4.009147065140000298E-51, 1.000000000000000000 ) ) ;
#12878=CIRCLE ( 'NONE', #22381, 9.000000000000000000 ) ;
#12889=LINE ( 'NONE', #14803, #8184 ) ;
#12906=FACE_OUTER_BOUND ( 'NONE', #5901, .T. ) ;
#12920=ORIENTED_EDGE ( 'NONE', *, *, #1695, .T. ) ;
#12956=LINE ( 'NONE', #21669, #23031 ) ;
#12990=FACE_OUTER_BOUND ( 'NONE', #6165, .T. ) ;
#13018=EDGE_CURVE ( 'NONE', #9539, #11240, #4288, .T. ) ;
#13039=DIRECTION ( 'NONE',  ( 0.000000000000000000, -1.000000000000000000, 0.000000000000000000 ) ) ;
#13064=ORIENTED_EDGE ( 'NONE', *, *, #6985, .T. ) ;
#13147=AXIS2_PLACEMENT_3D ( 'NONE', #3018, #21102, #12158 ) ;
#13150=ADVANCED_FACE ( 'NONE', ( #21061 ), #4636, .F. ) ;
#13160=FACE_OUTER_BOUND ( 'NONE', #19473, .T. ) ;
#13161=ORIENTED_EDGE ( 'NONE', *, *, #5935, .F. ) ;
#13168=CARTESIAN_POINT ( 'NONE',  ( 12.50000000010000001, 16.89444872450000190, -143.5552959529999839 ) ) ;
#13195=CARTESIAN_POINT ( 'NONE',  ( 0.5000000001590285681, 16.89444872450000190, -139.5552959529864268 ) ) ;
#13200=CARTESIAN_POINT ( 'NONE',  ( 0.5000000001659999915, 20.50000000000000000, -136.5552959530000123 ) ) ;
#13283=AXIS2_PLACEMENT_3D ( 'NONE', #6852, #21149, #13635 ) ;
#13290=EDGE_LOOP ( 'NONE', ( #21870, #4748, #12508, #23242 ) ) ;
#13292=ADVANCED_FACE ( 'NONE', ( #19621 ), #18069, .F. ) ;
#13324=LINE ( 'NONE', #16782, #13998 ) ;
#13340=CLOSED_SHELL ( 'NONE', ( #4891, #665, #10544, #21452, #10527, #14059, #15153, #13292, #5179, #18694, #22768, #14670, #21211, #15936, #22088, #4109, #11223, #2540, #13150, #7327, #9649, #19380, #22044, #9078, #1692, #8655, #17987, #2013, #18333, #9874 ) ) ;
#13353=CARTESIAN_POINT ( 'NONE',  ( -2.499999999859999988, 31.00000000000000000, -147.5552959529999839 ) ) ;
#13395=CARTESIAN_POINT ( 'NONE',  ( 1.000000000140000012, 36.50000000000000000, -147.0552959529999839 ) ) ;
#13417=CARTESIAN_POINT ( 'NONE',  ( 0.5000000001409999895, 20.50000000000000000, -147.5552959529999839 ) ) ;
#13425=EDGE_LOOP ( 'NONE', ( #705, #7669, #13161, #15354 ) ) ;
#13471=LINE ( 'NONE', #762, #15042 ) ;
#13544=CARTESIAN_POINT ( 'NONE',  ( 2.500000000170000014, 24.50000000000000000, -136.5552959530000123 ) ) ;
#13550=DIRECTION ( 'NONE',  ( 0.000000000000000000, 1.000000000000000000, 0.000000000000000000 ) ) ;
#13589=DIRECTION ( 'NONE',  ( 0.000000000000000000, 1.000000000000000000, 0.000000000000000000 ) ) ;
#13635=DIRECTION ( 'NONE',  ( 1.000000000000000000, 0.000000000000000000, -2.259303855112193156E-12 ) ) ;
#13641=CARTESIAN_POINT ( 'NONE',  ( 6.500000000159999125, 20.50000000000000000, -139.5552959529999839 ) ) ;
#13652=CYLINDRICAL_SURFACE ( 'NONE', #5369, 8.000000000000000000 ) ;
#13675=LINE ( 'NONE', #20949, #1121 ) ;
#13681=CIRCLE ( 'NONE', #13283, 5.000000000000000888 ) ;
#13709=CARTESIAN_POINT ( 'NONE',  ( 2.500000000130000011, 20.50000000000000000, -150.5552959529999839 ) ) ;
#13710=LINE ( 'NONE', #12268, #20507 ) ;
#13772=DIRECTION ( 'NONE',  ( 0.000000000000000000, 1.000000000000000000, 0.000000000000000000 ) ) ;
#13774=DIRECTION ( 'NONE',  ( -1.000000000000000000, 0.000000000000000000, 2.259525899719999991E-12 ) ) ;
#13783=DIRECTION ( 'NONE',  ( 2.257144641399999941E-12, -4.009147065136860232E-51, 1.000000000000000000 ) ) ;
#13785=DIRECTION ( 'NONE',  ( -2.257115129720000004E-12, 0.000000000000000000, -1.000000000000000000 ) ) ;
#13790=ORIENTED_EDGE ( 'NONE', *, *, #20162, .T. ) ;
#13798=EDGE_LOOP ( 'NONE', ( #10786, #3063, #21761, #39 ) ) ;
#13832=( NAMED_UNIT ( * ) SI_UNIT ( $, .STERADIAN. ) SOLID_ANGLE_UNIT ( ) );
#13907=CARTESIAN_POINT ( 'NONE',  ( 6.000000000160000013, 41.50000000000000000, -140.5552959529999839 ) ) ;
#13959=AXIS2_PLACEMENT_3D ( 'NONE', #13993, #23284, #21390 ) ;
#13965=CARTESIAN_POINT ( 'NONE',  ( -2.499999999859999988, 20.50000000000000000, -146.5552959529999839 ) ) ;
#13993=CARTESIAN_POINT ( 'NONE',  ( 1.000000000160000013, 36.50000000000000000, -140.5552959529999839 ) ) ;
#13998=VECTOR ( 'NONE', #7730, 1000.000000000000000 ) ;
#14018=( NAMED_UNIT ( * ) SI_UNIT ( $, .STERADIAN. ) SOLID_ANGLE_UNIT ( ) );
#14045=CARTESIAN_POINT ( 'NONE',  ( -2.499999999859999988, 41.50000000000000000, -147.5552959529999839 ) ) ;
#14049=DIRECTION ( 'NONE',  ( 0.000000000000000000, 1.000000000000000000, 0.000000000000000000 ) ) ;
#14053=EDGE_CURVE ( 'NONE', #8946, #21893, #18448, .T. ) ;
#14059=ADVANCED_FACE ( 'NONE', ( #8076 ), #6071, .T. ) ;
#14068=CARTESIAN_POINT ( 'NONE',  ( 6.000000000160000013, 36.50000000000000000, -140.0552959529999839 ) ) ;
#14072=FACE_OUTER_BOUND ( 'NONE', #13290, .T. ) ;
#14076=DIRECTION ( 'NONE',  ( 2.257144641399999941E-12, -4.009147065140000298E-51, 1.000000000000000000 ) ) ;
#14083=AXIS2_PLACEMENT_3D ( 'NONE', #3762, #3648, #7215 ) ;
#14086=ORIENTED_EDGE ( 'NONE', *, *, #4224, .T. ) ;
#14092=DIRECTION ( 'NONE',  ( -2.257146850379999957E-12, 0.000000000000000000, -1.000000000000000000 ) ) ;
#14118=VERTEX_POINT ( 'NONE', #11176 ) ;
#14146=( NAMED_UNIT ( * ) PLANE_ANGLE_UNIT ( ) SI_UNIT ( $, .RADIAN. ) );
#14157=ORIENTED_EDGE ( 'NONE', *, *, #11548, .T. ) ;
#14167=PLANE ( 'NONE',  #15966 ) ;
#14185=CARTESIAN_POINT ( 'NONE',  ( 6.000000000160000013, 29.48610037779999971, -139.5552959529999839 ) ) ;
#14199=( GEOMETRIC_REPRESENTATION_CONTEXT ( 3 ) GLOBAL_UNCERTAINTY_ASSIGNED_CONTEXT ( ( #12542 ) ) GLOBAL_UNIT_ASSIGNED_CONTEXT ( ( #8176, #12458, #14018 ) ) REPRESENTATION_CONTEXT ( 'NONE', 'WORKASPACE' ) );
#14239=CARTESIAN_POINT ( 'NONE',  ( -0.7499999998570000548, 41.50000000000000000, -146.5552959529999839 ) ) ;
#14241=CARTESIAN_POINT ( 'NONE',  ( 10.50000000010000001, 16.50000000000000000, -150.5552959529999839 ) ) ;
#14245=DIRECTION ( 'NONE',  ( 1.000000000000000000, 0.000000000000000000, -2.256131789327550371E-12 ) ) ;
#14249=ORIENTED_EDGE ( 'NONE', *, *, #4950, .T. ) ;
#14259=SURFACE_SIDE_STYLE ('',( #16045 ) ) ;
#14324=EDGE_CURVE ( 'NONE', #9455, #2716, #22717, .T. ) ;
#14327=FACE_OUTER_BOUND ( 'NONE', #12335, .T. ) ;
#14338=VERTEX_POINT ( 'NONE', #6413 ) ;
#14345=EDGE_CURVE ( 'NONE', #10310, #11694, #13675, .T. ) ;
#14389=CARTESIAN_POINT ( 'NONE',  ( 10.50000000020000002, 16.50000000000000000, -136.5552959530000123 ) ) ;
#14404=LINE ( 'NONE', #21681, #19828 ) ;
#14413=VERTEX_POINT ( 'NONE', #11036 ) ;
#14421=VECTOR ( 'NONE', #16257, 1000.000000000000000 ) ;
#14465=ORIENTED_EDGE ( 'NONE', *, *, #15044, .T. ) ;
#14484=FACE_OUTER_BOUND ( 'NONE', #21418, .T. ) ;
#14502=ORIENTED_EDGE ( 'NONE', *, *, #20666, .F. ) ;
#14530=VECTOR ( 'NONE', #16160, 1000.000000000000000 ) ;
#14542=ORIENTED_EDGE ( 'NONE', *, *, #1588, .F. ) ;
#14545=EDGE_LOOP ( 'NONE', ( #20316, #2005, #436, #1201, #21257 ) ) ;
#14581=VERTEX_POINT ( 'NONE', #9471 ) ;
#14606=VECTOR ( 'NONE', #20406, 1000.000000000000000 ) ;
#14608=EDGE_CURVE ( 'NONE', #3481, #21363, #18969, .T. ) ;
#14621=EDGE_CURVE ( 'NONE', #11240, #11694, #2824, .T. ) ;
#14635=CARTESIAN_POINT ( 'NONE',  ( 12.50000000020000002, 20.50000000000000000, -139.5552959529999839 ) ) ;
#14654=LINE ( 'NONE', #7394, #18093 ) ;
#14670=ADVANCED_FACE ( 'NONE', ( #9775, #18958 ), #418, .T. ) ;
#14685=ORIENTED_EDGE ( 'NONE', *, *, #15873, .F. ) ;
#14686=VECTOR ( 'NONE', #19156, 1000.000000000000000 ) ;
#14701=AXIS2_PLACEMENT_3D ( 'NONE', #2665, #15384, #999 ) ;
#14706=ORIENTED_EDGE ( 'NONE', *, *, #13018, .T. ) ;
#14713=ORIENTED_EDGE ( 'NONE', *, *, #20439, .F. ) ;
#14719=CIRCLE ( 'NONE', #13959, 5.000000000000000888 ) ;
#14724=EDGE_CURVE ( 'NONE', #14338, #20751, #19301, .T. ) ;
#14742=DIRECTION ( 'NONE',  ( 2.257305453670000045E-12, 0.000000000000000000, 1.000000000000000000 ) ) ;
#14745=CARTESIAN_POINT ( 'NONE',  ( 6.500000000159999125, 20.50000000000000000, -140.5552959529999839 ) ) ;
#14763=EDGE_CURVE ( 'NONE', #10310, #14581, #13710, .T. ) ;
#14780=AXIS2_PLACEMENT_3D ( 'NONE', #4172, #2285, #18798 ) ;
#14803=CARTESIAN_POINT ( 'NONE',  ( 6.000000000140000012, 36.50000000000000000, -147.0552959529999839 ) ) ;
#14811=EDGE_LOOP ( 'NONE', ( #9030, #6221, #9957, #439 ) ) ;
#14822=EDGE_LOOP ( 'NONE', ( #55, #17616 ) ) ;
#14923=CARTESIAN_POINT ( 'NONE',  ( -2.499999999839999987, 20.50000000000000000, -140.5552959529999839 ) ) ;
#14928=ORIENTED_EDGE ( 'NONE', *, *, #5010, .T. ) ;
#14985=EDGE_LOOP ( 'NONE', ( #18512, #12230, #12543, #9389 ) ) ;
#15038=ORIENTED_EDGE ( 'NONE', *, *, #14608, .T. ) ;
#15042=VECTOR ( 'NONE', #13589, 1000.000000000000000 ) ;
#15044=EDGE_CURVE ( 'NONE', #9795, #11233, #7927, .T. ) ;
#15052=CARTESIAN_POINT ( 'NONE',  ( -2.499999999859999988, 20.50000000000000000, -147.0552959529999839 ) ) ;
#15061=DIRECTION ( 'NONE',  ( 2.257749542879999954E-12, 0.000000000000000000, 1.000000000000000000 ) ) ;
#15119=ORIENTED_EDGE ( 'NONE', *, *, #11527, .F. ) ;
#15153=ADVANCED_FACE ( 'NONE', ( #14484 ), #5548, .T. ) ;
#15175=EDGE_CURVE ( 'NONE', #2933, #17870, #22254, .T. ) ;
#15203=AXIS2_PLACEMENT_3D ( 'NONE', #13395, #20321, #20665 ) ;
#15211=DIRECTION ( 'NONE',  ( 0.000000000000000000, -1.000000000000000000, 0.000000000000000000 ) ) ;
#15234=DIRECTION ( 'NONE',  ( 0.000000000000000000, -1.000000000000000000, 0.000000000000000000 ) ) ;
#15267=FILL_AREA_STYLE ('',( #7987 ) ) ;
#15296=EDGE_CURVE ( 'NONE', #18780, #10634, #4463, .T. ) ;
#15354=ORIENTED_EDGE ( 'NONE', *, *, #12736, .F. ) ;
#15384=DIRECTION ( 'NONE',  ( 2.257144641399999941E-12, -4.009147065140000298E-51, 1.000000000000000000 ) ) ;
#15396=CARTESIAN_POINT ( 'NONE',  ( 0.5000000001500000124, 24.10555127549999810, -143.5552959529999839 ) ) ;
#15417=CARTESIAN_POINT ( 'NONE',  ( 6.500000000170000014, 20.50000000000000000, -136.5552959530000123 ) ) ;
#15431=CIRCLE ( 'NONE', #5170, 7.000000000000000888 ) ;
#15479=AXIS2_PLACEMENT_3D ( 'NONE', #21665, #20339, #2034 ) ;
#15559=DIRECTION ( 'NONE',  ( 2.257144641399999941E-12, 0.000000000000000000, 1.000000000000000000 ) ) ;
#15573=VECTOR ( 'NONE', #19113, 1000.000000000000000 ) ;
#15619=EDGE_CURVE ( 'NONE', #3677, #12862, #21128, .T. ) ;
#15648=EDGE_CURVE ( 'NONE', #9722, #2716, #12889, .T. ) ;
#15665=FACE_OUTER_BOUND ( 'NONE', #10002, .T. ) ;
#15705=( GEOMETRIC_REPRESENTATION_CONTEXT ( 3 ) GLOBAL_UNCERTAINTY_ASSIGNED_CONTEXT ( ( #182 ) ) GLOBAL_UNIT_ASSIGNED_CONTEXT ( ( #19737, #14146, #15920 ) ) REPRESENTATION_CONTEXT ( 'NONE', 'WORKASPACE' ) );
#15740=CARTESIAN_POINT ( 'NONE',  ( 6.500000000140000012, 20.50000000000000000, -146.5552959529999839 ) ) ;
#15757=CARTESIAN_POINT ( 'NONE',  ( 6.000000000160000013, 29.48610037779999971, -140.5552959529999839 ) ) ;
#15784=ORIENTED_EDGE ( 'NONE', *, *, #10078, .F. ) ;
#15822=AXIS2_PLACEMENT_3D ( 'NONE', #21244, #23140, #6709 ) ;
#15847=DIRECTION ( 'NONE',  ( 1.000000000000000000, 0.000000000000000000, -2.256131789327549967E-12 ) ) ;
#15872=CARTESIAN_POINT ( 'NONE',  ( 6.000000000140000012, 41.50000000000000000, -147.5552959529999839 ) ) ;
#15873=EDGE_CURVE ( 'NONE', #10865, #20660, #13471, .T. ) ;
#15891=ORIENTED_EDGE ( 'NONE', *, *, #16514, .F. ) ;
#15892=LINE ( 'NONE', #3758, #14421 ) ;
#15920=( NAMED_UNIT ( * ) SI_UNIT ( $, .STERADIAN. ) SOLID_ANGLE_UNIT ( ) );
#15936=ADVANCED_FACE ( 'NONE', ( #14072 ), #10475, .F. ) ;
#15966=AXIS2_PLACEMENT_3D ( 'NONE', #14045, #2869, #10103 ) ;
#16015=CARTESIAN_POINT ( 'NONE',  ( 1.000000000160000013, 41.50000000000000000, -140.5552959529999839 ) ) ;
#16045=SURFACE_STYLE_FILL_AREA ( #10547 ) ;
#16090=EDGE_CURVE ( 'NONE', #18121, #10865, #15431, .T. ) ;
#16093=CARTESIAN_POINT ( 'NONE',  ( 6.000000000160000013, 29.48610037779999971, -140.0552959529999839 ) ) ;
#16129=EDGE_CURVE ( 'NONE', #2164, #9556, #14654, .T. ) ;
#16133=ORIENTED_EDGE ( 'NONE', *, *, #14763, .T. ) ;
#16160=DIRECTION ( 'NONE',  ( 1.000000000000000000, 0.000000000000000000, -2.255973186040000320E-12 ) ) ;
#16180=DIRECTION ( 'NONE',  ( 0.000000000000000000, -1.000000000000000000, 0.000000000000000000 ) ) ;
#16222=ORIENTED_EDGE ( 'NONE', *, *, #14324, .F. ) ;
#16257=DIRECTION ( 'NONE',  ( 2.257157423930000049E-12, 0.000000000000000000, 1.000000000000000000 ) ) ;
#16277=LINE ( 'NONE', #12102, #10328 ) ;
#16320=EDGE_CURVE ( 'NONE', #21917, #2716, #21871, .T. ) ;
#16402=PRODUCT_CONTEXT ( 'NONE', #2653, 'mechanical' ) ;
#16434=DIRECTION ( 'NONE',  ( 1.000000000000000000, 0.000000000000000000, -2.257144641399999941E-12 ) ) ;
#16492=LINE ( 'NONE', #21971, #12042 ) ;
#16514=EDGE_CURVE ( 'NONE', #8221, #3481, #19629, .T. ) ;
#16617=SHAPE_DEFINITION_REPRESENTATION ( #9976, #17559 ) ;
#16626=DIRECTION ( 'NONE',  ( 2.257144641404620116E-12, 2.777754792983395132E-24, 1.000000000000000000 ) ) ;
#16637=CARTESIAN_POINT ( 'NONE',  ( 1.000000000140000012, 41.50000000000000000, -146.5552959529999839 ) ) ;
#16654=VECTOR ( 'NONE', #15061, 1000.000000000000000 ) ;
#16658=EDGE_LOOP ( 'NONE', ( #1232, #1491, #13064, #17178 ) ) ;
#16699=DIRECTION ( 'NONE',  ( 1.000000000000000000, 0.000000000000000000, -2.257453483404484831E-12 ) ) ;
#16722=CARTESIAN_POINT ( 'NONE',  ( 6.500000000149999124, 20.50000000000000000, -143.5552959529999839 ) ) ;
#16744=LINE ( 'NONE', #13168, #10947 ) ;
#16782=CARTESIAN_POINT ( 'NONE',  ( 6.000000000140000012, 32.99305018889999275, -147.5552959529999839 ) ) ;
#16783=ORIENTED_EDGE ( 'NONE', *, *, #21236, .F. ) ;
#16794=VECTOR ( 'NONE', #8367, 1000.000000000000000 ) ;
#16796=VECTOR ( 'NONE', #8332, 1000.000000000000000 ) ;
#16843=EDGE_CURVE ( 'NONE', #9722, #6969, #19201, .T. ) ;
#16916=CARTESIAN_POINT ( 'NONE',  ( -2.499999999839999987, 41.50000000000000000, -140.5552959529999839 ) ) ;
#17014=CARTESIAN_POINT ( 'NONE',  ( 1.000000000140000012, 36.50000000000000000, -146.5552959529999839 ) ) ;
#17036=SURFACE_SIDE_STYLE ('',( #22747 ) ) ;
#17084=DIRECTION ( 'NONE',  ( 0.000000000000000000, 0.000000000000000000, 1.000000000000000000 ) ) ;
#17176=CARTESIAN_POINT ( 'NONE',  ( 6.500000000170000014, 20.50000000000000000, -136.5552959530000123 ) ) ;
#17178=ORIENTED_EDGE ( 'NONE', *, *, #14608, .F. ) ;
#17200=ORIENTED_EDGE ( 'NONE', *, *, #5032, .T. ) ;
#17211=DIRECTION ( 'NONE',  ( 2.257144641399999941E-12, -4.009147065136860232E-51, 1.000000000000000000 ) ) ;
#17223=ORIENTED_EDGE ( 'NONE', *, *, #14345, .F. ) ;
#17225=COLOUR_RGB ( '', 0.31764706, 0.68627451, 0.89019608) ;
#17280=DIRECTION ( 'NONE',  ( 0.000000000000000000, 1.000000000000000000, 0.000000000000000000 ) ) ;
#17282=LINE ( 'NONE', #6220, #8700 ) ;
#17287=DIRECTION ( 'NONE',  ( 0.8571428571427679444, 0.5150787536378610421, -1.934960128632415569E-12 ) ) ;
#17340=CARTESIAN_POINT ( 'NONE',  ( 6.500000000159999125, 20.50000000000000000, -140.0552959529999839 ) ) ;
#17342=CARTESIAN_POINT ( 'NONE',  ( 10.50000000010000001, 16.50000000000000000, -143.5552959529999839 ) ) ;
#17345=VERTEX_POINT ( 'NONE', #7739 ) ;
#17387=CARTESIAN_POINT ( 'NONE',  ( 6.500000000170000014, 24.50000000000000000, -136.5552959530000123 ) ) ;
#17449=DIRECTION ( 'NONE',  ( 2.257144641399999941E-12, -4.009147065140000298E-51, 1.000000000000000000 ) ) ;
#17455=VECTOR ( 'NONE', #13774, 1000.000000000000000 ) ;
#17460=DIRECTION ( 'NONE',  ( 0.000000000000000000, 1.000000000000000000, 0.000000000000000000 ) ) ;
#17482=CARTESIAN_POINT ( 'NONE',  ( 12.50000000020000002, 16.89444872450000190, -136.5552959530000123 ) ) ;
#17489=LINE ( 'NONE', #10215, #14686 ) ;
#17500=LINE ( 'NONE', #23093, #4137 ) ;
#17505=DIRECTION ( 'NONE',  ( 2.257083409060000051E-12, 0.000000000000000000, 1.000000000000000000 ) ) ;
#17508=( GEOMETRIC_REPRESENTATION_CONTEXT ( 3 ) GLOBAL_UNCERTAINTY_ASSIGNED_CONTEXT ( ( #10399 ) ) GLOBAL_UNIT_ASSIGNED_CONTEXT ( ( #6218, #20734, #13832 ) ) REPRESENTATION_CONTEXT ( 'NONE', 'WORKASPACE' ) );
#17529=CIRCLE ( 'NONE', #7272, 6.999999999999999112 ) ;
#17559=SHAPE_REPRESENTATION ( 'Spindle Hub', ( #5025 ), #14199 ) ;
#17568=VERTEX_POINT ( 'NONE', #5584 ) ;
#17593=CARTESIAN_POINT ( 'NONE',  ( 0.5000000001340000333, 16.89444872450000190, -150.5552959529999839 ) ) ;
#17616=ORIENTED_EDGE ( 'NONE', *, *, #8288, .T. ) ;
#17630=ORIENTED_EDGE ( 'NONE', *, *, #6985, .F. ) ;
#17641=EDGE_CURVE ( 'NONE', #2758, #14118, #12956, .T. ) ;
#17649=AXIS2_PLACEMENT_3D ( 'NONE', #20877, #20526, #7775 ) ;
#17704=LINE ( 'NONE', #19378, #14530 ) ;
#17707=EDGE_CURVE ( 'NONE', #18121, #3881, #2493, .T. ) ;
#17771=CARTESIAN_POINT ( 'NONE',  ( 12.50000000010000001, 24.10555127549999810, -143.5552959529999839 ) ) ;
#17777=VECTOR ( 'NONE', #12320, 1000.000000000000000 ) ;
#17804=ORIENTED_EDGE ( 'NONE', *, *, #8331, .T. ) ;
#17870=VERTEX_POINT ( 'NONE', #4974 ) ;
#17894=ORIENTED_EDGE ( 'NONE', *, *, #4950, .F. ) ;
#17983=DIRECTION ( 'NONE',  ( 2.257144641399999941E-12, -4.009147065140000298E-51, 1.000000000000000000 ) ) ;
#17987=ADVANCED_FACE ( 'NONE', ( #6519, #4736 ), #11980, .F. ) ;
#17993=ORIENTED_EDGE ( 'NONE', *, *, #19396, .F. ) ;
#18021=LINE ( 'NONE', #8720, #20158 ) ;
#18041=CARTESIAN_POINT ( 'NONE',  ( 2.500000000170000014, 16.50000000000000000, -136.5552959530000123 ) ) ;
#18069=PLANE ( 'NONE',  #12628 ) ;
#18093=VECTOR ( 'NONE', #21925, 1000.000000000000000 ) ;
#18095=DIRECTION ( 'NONE',  ( 0.000000000000000000, 1.000000000000000000, 0.000000000000000000 ) ) ;
#18107=EDGE_LOOP ( 'NONE', ( #6813, #20621, #14086, #9210 ) ) ;
#18121=VERTEX_POINT ( 'NONE', #8718 ) ;
#18128=ORIENTED_EDGE ( 'NONE', *, *, #11548, .F. ) ;
#18140=EDGE_CURVE ( 'NONE', #20358, #14413, #9347, .T. ) ;
#18173=CARTESIAN_POINT ( 'NONE',  ( -2.499999999839999987, 20.50000000000000000, -140.0552959529999839 ) ) ;
#18181=FILL_AREA_STYLE_COLOUR ( '', #17225 ) ;
#18193=LINE ( 'NONE', #1788, #12478 ) ;
#18286=COLOUR_RGB ( '', 0.31764706, 0.68627451, 0.89019608) ;
#18291=DIRECTION ( 'NONE',  ( -0.8571428571427679444, -0.5150787536378610421, 1.934960128632415569E-12 ) ) ;
#18295=ORIENTED_EDGE ( 'NONE', *, *, #16843, .T. ) ;
#18303=ORIENTED_EDGE ( 'NONE', *, *, #19941, .T. ) ;
#18333=ADVANCED_FACE ( 'NONE', ( #14327 ), #18370, .F. ) ;
#18345=ADVANCED_BREP_SHAPE_REPRESENTATION ( '', ( #11693, #5025 ), #14199 ) ;
#18370=PLANE ( 'NONE',  #21922 ) ;
#18423=CYLINDRICAL_SURFACE ( 'NONE', #10566, 7.000000000000000888 ) ;
#18448=LINE ( 'NONE', #13200, #5649 ) ;
#18512=ORIENTED_EDGE ( 'NONE', *, *, #17707, .T. ) ;
#18539=PLANE ( 'NONE',  #15479 ) ;
#18549=EDGE_CURVE ( 'NONE', #20660, #3881, #8965, .T. ) ;
#18564=EDGE_CURVE ( 'NONE', #8517, #18121, #17489, .T. ) ;
#18656=ORIENTED_EDGE ( 'NONE', *, *, #12222, .F. ) ;
#18694=ADVANCED_FACE ( 'NONE', ( #2 ), #8657, .F. ) ;
#18780=VERTEX_POINT ( 'NONE', #1565 ) ;
#18798=DIRECTION ( 'NONE',  ( -2.257144641399999941E-12, 0.000000000000000000, -1.000000000000000000 ) ) ;
#18815=VECTOR ( 'NONE', #16180, 1000.000000000000000 ) ;
#18869=DIRECTION ( 'NONE',  ( 2.257144641399999941E-12, -4.009147065140000298E-51, 1.000000000000000000 ) ) ;
#18878=CYLINDRICAL_SURFACE ( 'NONE', #6273, 8.000000000000000000 ) ;
#18909=CARTESIAN_POINT ( 'NONE',  ( -2.499999999839999987, 20.50000000000000000, -139.5552959529999839 ) ) ;
#18958=FACE_OUTER_BOUND ( 'NONE', #22545, .T. ) ;
#18959=VECTOR ( 'NONE', #23429, 1000.000000000000000 ) ;
#18961=AXIS2_PLACEMENT_3D ( 'NONE', #5496, #4795, #17287 ) ;
#18969=CIRCLE ( 'NONE', #7559, 9.000000000000000000 ) ;
#18992=DIRECTION ( 'NONE',  ( 1.000000000000000000, 0.000000000000000000, -2.256131789327549967E-12 ) ) ;
#19003=CIRCLE ( 'NONE', #4565, 7.000000000000000000 ) ;
#19004=AXIS2_PLACEMENT_3D ( 'NONE', #20299, #6119, #547 ) ;
#19016=VECTOR ( 'NONE', #22709, 1000.000000000000000 ) ;
#19033=CARTESIAN_POINT ( 'NONE',  ( 6.000000000140000012, 32.99305018889999275, -146.5552959529999839 ) ) ;
#19081=EDGE_CURVE ( 'NONE', #21363, #20751, #5062, .T. ) ;
#19109=EDGE_LOOP ( 'NONE', ( #6354, #20458, #13790, #15891 ) ) ;
#19113=DIRECTION ( 'NONE',  ( 2.257146850379999957E-12, 0.000000000000000000, 1.000000000000000000 ) ) ;
#19156=DIRECTION ( 'NONE',  ( 2.257146850379999957E-12, 0.000000000000000000, 1.000000000000000000 ) ) ;
#19167=ORIENTED_EDGE ( 'NONE', *, *, #21530, .F. ) ;
#19179=PRESENTATION_STYLE_ASSIGNMENT (( #6328 ) ) ;
#19201=CIRCLE ( 'NONE', #3636, 5.000000000000000000 ) ;
#19244=CARTESIAN_POINT ( 'NONE',  ( 6.500000000140000012, 20.50000000000000000, -147.5552959529999839 ) ) ;
#19283=CARTESIAN_POINT ( 'NONE',  ( 12.50000000009097079, 24.10555127549999810, -147.5552959530157864 ) ) ;
#19301=LINE ( 'NONE', #14068, #8326 ) ;
#19323=EDGE_LOOP ( 'NONE', ( #6621, #17223, #16133, #18303 ) ) ;
#19332=EDGE_CURVE ( 'NONE', #9556, #8221, #7996, .T. ) ;
#19339=CIRCLE ( 'NONE', #10204, 7.000000000000000888 ) ;
#19343=AXIS2_PLACEMENT_3D ( 'NONE', #3697, #17983, #16434 ) ;
#19344=EDGE_LOOP ( 'NONE', ( #17993, #17894 ) ) ;
#19378=CARTESIAN_POINT ( 'NONE',  ( 6.500000000130000011, 24.50000000000000000, -150.5552959529999839 ) ) ;
#19380=ADVANCED_FACE ( 'NONE', ( #4440 ), #7652, .F. ) ;
#19395=DIRECTION ( 'NONE',  ( -2.257146850379999957E-12, 0.000000000000000000, -1.000000000000000000 ) ) ;
#19396=EDGE_CURVE ( 'NONE', #5071, #10763, #22697, .T. ) ;
#19415=CARTESIAN_POINT ( 'NONE',  ( 10.50000000010000001, 24.50000000000000000, -150.5552959529999839 ) ) ;
#19473=EDGE_LOOP ( 'NONE', ( #19940, #4622, #18295, #23155 ) ) ;
#19578=DIRECTION ( 'NONE',  ( 0.000000000000000000, 1.000000000000000000, 0.000000000000000000 ) ) ;
#19621=FACE_OUTER_BOUND ( 'NONE', #11493, .T. ) ;
#19629=LINE ( 'NONE', #1915, #18815 ) ;
#19737=( LENGTH_UNIT ( ) NAMED_UNIT ( * ) SI_UNIT ( .MILLI., .METRE. ) );
#19771=FACE_BOUND ( 'NONE', #19344, .T. ) ;
#19795=ORIENTED_EDGE ( 'NONE', *, *, #10262, .F. ) ;
#19803=ORIENTED_EDGE ( 'NONE', *, *, #3888, .F. ) ;
#19828=VECTOR ( 'NONE', #18095, 1000.000000000000000 ) ;
#19839=DIRECTION ( 'NONE',  ( 2.257144641399999941E-12, -4.009147065140000298E-51, 1.000000000000000000 ) ) ;
#19923=DIRECTION ( 'NONE',  ( -2.257144641399999941E-12, 0.000000000000000000, -1.000000000000000000 ) ) ;
#19940=ORIENTED_EDGE ( 'NONE', *, *, #16320, .T. ) ;
#19941=EDGE_CURVE ( 'NONE', #14581, #11240, #4620, .T. ) ;
#19966=SURFACE_STYLE_USAGE ( .BOTH. , #14259 ) ;
#20036=LINE ( 'NONE', #17771, #20518 ) ;
#20148=PLANE ( 'NONE',  #23253 ) ;
#20158=VECTOR ( 'NONE', #4819, 1000.000000000000000 ) ;
#20162=EDGE_CURVE ( 'NONE', #9674, #3481, #20201, .T. ) ;
#20187=PLANE ( 'NONE',  #19004 ) ;
#20192=VECTOR ( 'NONE', #17280, 1000.000000000000000 ) ;
#20201=LINE ( 'NONE', #18173, #16654 ) ;
#20299=CARTESIAN_POINT ( 'NONE',  ( 10.50000000020000002, 24.50000000000000000, -136.5552959530000123 ) ) ;
#20316=ORIENTED_EDGE ( 'NONE', *, *, #4229, .T. ) ;
#20321=DIRECTION ( 'NONE',  ( 2.257144641399999941E-12, 0.000000000000000000, 1.000000000000000000 ) ) ;
#20339=DIRECTION ( 'NONE',  ( 2.257144641399999941E-12, -4.009147065140000298E-51, 1.000000000000000000 ) ) ;
#20358=VERTEX_POINT ( 'NONE', #1028 ) ;
#20369=AXIS2_PLACEMENT_3D ( 'NONE', #7441, #312, #8984 ) ;
#20399=AXIS2_PLACEMENT_3D ( 'NONE', #14389, #3567, #5222 ) ;
#20406=DIRECTION ( 'NONE',  ( 2.257115129720000004E-12, 0.000000000000000000, 1.000000000000000000 ) ) ;
#20429=CYLINDRICAL_SURFACE ( 'NONE', #15203, 5.000000000000000000 ) ;
#20432=ORIENTED_EDGE ( 'NONE', *, *, #6474, .F. ) ;
#20439=EDGE_CURVE ( 'NONE', #18780, #17568, #12073, .T. ) ;
#20458=ORIENTED_EDGE ( 'NONE', *, *, #8716, .T. ) ;
#20459=CARTESIAN_POINT ( 'NONE',  ( 12.50000000010000001, 16.89444872450000190, -150.5552959529999839 ) ) ;
#20507=VECTOR ( 'NONE', #22882, 1000.000000000000000 ) ;
#20518=VECTOR ( 'NONE', #21591, 1000.000000000000000 ) ;
#20526=DIRECTION ( 'NONE',  ( 3.882490197650000213E-51, -1.000000000000000000, -4.009147065150000317E-51 ) ) ;
#20621=ORIENTED_EDGE ( 'NONE', *, *, #14724, .F. ) ;
#20660=VERTEX_POINT ( 'NONE', #19283 ) ;
#20665=DIRECTION ( 'NONE',  ( 1.000000000000000000, 0.000000000000000000, -2.259303855112193560E-12 ) ) ;
#20666=EDGE_CURVE ( 'NONE', #8429, #2933, #17500, .T. ) ;
#20686=ORIENTED_EDGE ( 'NONE', *, *, #21184, .F. ) ;
#20734=( NAMED_UNIT ( * ) PLANE_ANGLE_UNIT ( ) SI_UNIT ( $, .RADIAN. ) );
#20751=VERTEX_POINT ( 'NONE', #10570 ) ;
#20877=CARTESIAN_POINT ( 'NONE',  ( -2.499999999839999987, 41.50000000000000000, -140.5552959529999839 ) ) ;
#20943=DIRECTION ( 'NONE',  ( -1.000000000000000000, 0.000000000000000000, 2.257453483404484831E-12 ) ) ;
#20949=CARTESIAN_POINT ( 'NONE',  ( 2.500000000150000012, 16.50000000000000000, -143.5552959529999839 ) ) ;
#20974=CYLINDRICAL_SURFACE ( 'NONE', #2744, 7.000000000000000888 ) ;
#21002=PLANE ( 'NONE',  #5338 ) ;
#21028=PRODUCT ( 'Spindle Hub', 'Spindle Hub', '', ( #16402 ) ) ;
#21029=CARTESIAN_POINT ( 'NONE',  ( 2.500000000130000011, 24.50000000000000000, -150.5552959529999839 ) ) ;
#21061=FACE_OUTER_BOUND ( 'NONE', #9809, .T. ) ;
#21067=FACE_OUTER_BOUND ( 'NONE', #8964, .T. ) ;
#21102=DIRECTION ( 'NONE',  ( -3.882490197650000213E-51, 1.000000000000000000, 4.009147065150000317E-51 ) ) ;
#21106=DIRECTION ( 'NONE',  ( 1.000000000000000000, 0.000000000000000000, -2.258609965721802837E-12 ) ) ;
#21128=LINE ( 'NONE', #12063, #12364 ) ;
#21149=DIRECTION ( 'NONE',  ( -2.257144641399999941E-12, 4.009147065140000298E-51, -1.000000000000000000 ) ) ;
#21184=EDGE_CURVE ( 'NONE', #9674, #1369, #12878, .T. ) ;
#21211=ADVANCED_FACE ( 'NONE', ( #15665 ), #6370, .F. ) ;
#21236=EDGE_CURVE ( 'NONE', #21893, #3677, #19339, .T. ) ;
#21244=CARTESIAN_POINT ( 'NONE',  ( 6.500000000159999125, 20.50000000000000000, -140.5552959529999839 ) ) ;
#21257=ORIENTED_EDGE ( 'NONE', *, *, #16320, .F. ) ;
#21363=VERTEX_POINT ( 'NONE', #14185 ) ;
#21368=DIRECTION ( 'NONE',  ( -1.000000000000000000, 1.190078432789999897E-50, 2.257144641399999941E-12 ) ) ;
#21390=DIRECTION ( 'NONE',  ( 1.000000000000000000, 0.000000000000000000, -2.259303855112193156E-12 ) ) ;
#21418=EDGE_LOOP ( 'NONE', ( #14465, #7960, #16783, #19795 ) ) ;
#21419=LINE ( 'NONE', #12592, #18959 ) ;
#21431=DIRECTION ( 'NONE',  ( 2.257144641399999941E-12, -4.009147065140000298E-51, 1.000000000000000000 ) ) ;
#21452=ADVANCED_FACE ( 'NONE', ( #35 ), #21812, .T. ) ;
#21489=EDGE_LOOP ( 'NONE', ( #23274, #8286, #14542, #23235 ) ) ;
#21530=EDGE_CURVE ( 'NONE', #10763, #14413, #6337, .T. ) ;
#21537=DIRECTION ( 'NONE',  ( 1.000000000000000000, 0.000000000000000000, -2.258609965721802837E-12 ) ) ;
#21553=CARTESIAN_POINT ( 'NONE',  ( -0.7499999998430000314, 41.50000000000000000, -140.5552959529999839 ) ) ;
#21591=DIRECTION ( 'NONE',  ( 2.257242012349999735E-12, 0.000000000000000000, 1.000000000000000000 ) ) ;
#21597=CARTESIAN_POINT ( 'NONE',  ( -2.499999999859999988, 20.50000000000000000, -147.5552959529999839 ) ) ;
#21619=ORIENTED_EDGE ( 'NONE', *, *, #8288, .F. ) ;
#21645=VERTEX_POINT ( 'NONE', #8442 ) ;
#21665=CARTESIAN_POINT ( 'NONE',  ( 6.500000000159999125, 20.50000000000000000, -140.5552959529999839 ) ) ;
#21669=CARTESIAN_POINT ( 'NONE',  ( -2.499999999859999988, 41.50000000000000000, -147.0552959529999839 ) ) ;
#21681=CARTESIAN_POINT ( 'NONE',  ( 6.000000000160000013, 32.99305018889999275, -140.5552959529999839 ) ) ;
#21761=ORIENTED_EDGE ( 'NONE', *, *, #21530, .T. ) ;
#21768=ORIENTED_EDGE ( 'NONE', *, *, #6735, .F. ) ;
#21812=CYLINDRICAL_SURFACE ( 'NONE', #18961, 7.000000000000000888 ) ;
#21870=ORIENTED_EDGE ( 'NONE', *, *, #23457, .T. ) ;
#21871=CIRCLE ( 'NONE', #4753, 5.000000000000000000 ) ;
#21888=DIRECTION ( 'NONE',  ( 2.257305453670000045E-12, 0.000000000000000000, 1.000000000000000000 ) ) ;
#21893=VERTEX_POINT ( 'NONE', #5111 ) ;
#21903=DIRECTION ( 'NONE',  ( 0.000000000000000000, 1.000000000000000000, 0.000000000000000000 ) ) ;
#21908=ORIENTED_EDGE ( 'NONE', *, *, #4224, .F. ) ;
#21917=VERTEX_POINT ( 'NONE', #16637 ) ;
#21922=AXIS2_PLACEMENT_3D ( 'NONE', #21597, #10740, #19923 ) ;
#21925=DIRECTION ( 'NONE',  ( 2.257083409060000051E-12, 0.000000000000000000, 1.000000000000000000 ) ) ;
#21971=CARTESIAN_POINT ( 'NONE',  ( 0.5000000001340000333, 20.50000000000000000, -150.5552959529999839 ) ) ;
#22002=ORIENTED_EDGE ( 'NONE', *, *, #19081, .F. ) ;
#22013=DIRECTION ( 'NONE',  ( 2.257144641399999941E-12, -4.009147065140000298E-51, 1.000000000000000000 ) ) ;
#22036=AXIS2_PLACEMENT_3D ( 'NONE', #14745, #22013, #1925 ) ;
#22044=ADVANCED_FACE ( 'NONE', ( #6164 ), #7934, .T. ) ;
#22062=ORIENTED_EDGE ( 'NONE', *, *, #15296, .T. ) ;
#22088=ADVANCED_FACE ( 'NONE', ( #22825 ), #13652, .T. ) ;
#22137=DIRECTION ( 'NONE',  ( 2.257749542879999954E-12, 0.000000000000000000, 1.000000000000000000 ) ) ;
#22172=LINE ( 'NONE', #13353, #11028 ) ;
#22174=EDGE_CURVE ( 'NONE', #17870, #3881, #7103, .T. ) ;
#22180=DIRECTION ( 'NONE',  ( 1.000000000000000000, -1.190078432789999897E-50, -2.257144641399999941E-12 ) ) ;
#22254=CIRCLE ( 'NONE', #20369, 7.000000000000000000 ) ;
#22288=ORIENTED_EDGE ( 'NONE', *, *, #11692, .T. ) ;
#22381=AXIS2_PLACEMENT_3D ( 'NONE', #6256, #18869, #11713 ) ;
#22450=STYLED_ITEM ( 'NONE', ( #19179 ), #11693 ) ;
#22545=EDGE_LOOP ( 'NONE', ( #9888, #7680, #295, #8481 ) ) ;
#22556=APPLICATION_CONTEXT ( 'automotive_design' ) ;
#22656=LINE ( 'NONE', #15396, #14606 ) ;
#22696=DIRECTION ( 'NONE',  ( -1.000000000000000000, 0.000000000000000000, 2.257453483404484831E-12 ) ) ;
#22697=CIRCLE ( 'NONE', #11288, 8.000000000000000000 ) ;
#22709=DIRECTION ( 'NONE',  ( 0.000000000000000000, -1.000000000000000000, 0.000000000000000000 ) ) ;
#22711=DIRECTION ( 'NONE',  ( 2.257144641399999941E-12, 0.000000000000000000, 1.000000000000000000 ) ) ;
#22717=LINE ( 'NONE', #19033, #10210 ) ;
#22747=SURFACE_STYLE_FILL_AREA ( #15267 ) ;
#22748=CIRCLE ( 'NONE', #9819, 8.000000000000000000 ) ;
#22768=ADVANCED_FACE ( 'NONE', ( #5731, #12990 ), #20148, .F. ) ;
#22803=DIRECTION ( 'NONE',  ( 1.190078432789999897E-50, 1.000000000000000000, 0.000000000000000000 ) ) ;
#22825=FACE_OUTER_BOUND ( 'NONE', #13798, .T. ) ;
#22872=CARTESIAN_POINT ( 'NONE',  ( 6.500000000149999124, 20.50000000000000000, -143.5552959529999839 ) ) ;
#22875=CARTESIAN_POINT ( 'NONE',  ( 12.50000000010000001, 16.89444872450000190, -147.5552959529999839 ) ) ;
#22882=DIRECTION ( 'NONE',  ( 1.000000000000000000, 0.000000000000000000, -2.259525899719999991E-12 ) ) ;
#22925=ORIENTED_EDGE ( 'NONE', *, *, #231, .F. ) ;
#22933=ORIENTED_EDGE ( 'NONE', *, *, #14345, .T. ) ;
#22941=CARTESIAN_POINT ( 'NONE',  ( 6.500000000130000011, 16.50000000000000000, -150.5552959529999839 ) ) ;
#23031=VECTOR ( 'NONE', #14742, 1000.000000000000000 ) ;
#23093=CARTESIAN_POINT ( 'NONE',  ( 12.50000000010000001, 20.50000000000000000, -150.5552959529999839 ) ) ;
#23128=CARTESIAN_POINT ( 'NONE',  ( 6.000000000140000012, 36.50000000000000000, -146.5552959529999839 ) ) ;
#23140=DIRECTION ( 'NONE',  ( 2.257144641399999941E-12, -4.009147065140000298E-51, 1.000000000000000000 ) ) ;
#23150=DIRECTION ( 'NONE',  ( 1.000000000000000000, 0.000000000000000000, -2.257453483404484831E-12 ) ) ;
#23155=ORIENTED_EDGE ( 'NONE', *, *, #12726, .T. ) ;
#23169=AXIS2_PLACEMENT_3D ( 'NONE', #15872, #21368, #23490 ) ;
#23221=AXIS2_PLACEMENT_3D ( 'NONE', #17340, #15559, #22696 ) ;
#23235=ORIENTED_EDGE ( 'NONE', *, *, #15175, .T. ) ;
#23242=ORIENTED_EDGE ( 'NONE', *, *, #1379, .T. ) ;
#23253=AXIS2_PLACEMENT_3D ( 'NONE', #6088, #12867, #4306 ) ;
#23256=VECTOR ( 'NONE', #17505, 1000.000000000000000 ) ;
#23274=ORIENTED_EDGE ( 'NONE', *, *, #22174, .T. ) ;
#23284=DIRECTION ( 'NONE',  ( 2.257144641399999941E-12, -4.009147065140000298E-51, 1.000000000000000000 ) ) ;
#23333=FACE_OUTER_BOUND ( 'NONE', #14545, .T. ) ;
#23334=FACE_OUTER_BOUND ( 'NONE', #4387, .T. ) ;
#23368=CARTESIAN_POINT ( 'NONE',  ( 6.500000000140000012, 28.50000000000000000, -146.5552959529999839 ) ) ;
#23377=EDGE_CURVE ( 'NONE', #14581, #21645, #16277, .T. ) ;
#23383=EDGE_LOOP ( 'NONE', ( #8998, #7915, #14713, #18128, #15784 ) ) ;
#23407=EDGE_LOOP ( 'NONE', ( #17804, #17200, #2341, #22925 ) ) ;
#23420=LINE ( 'NONE', #5210, #6450 ) ;
#23429=DIRECTION ( 'NONE',  ( 2.257242012349999735E-12, 0.000000000000000000, 1.000000000000000000 ) ) ;
#23457=EDGE_CURVE ( 'NONE', #10188, #9539, #17704, .T. ) ;
#23490=DIRECTION ( 'NONE',  ( 1.190078432789999897E-50, 1.000000000000000000, 0.000000000000000000 ) ) ;
#23494=DIRECTION ( 'NONE',  ( 1.000000000000000000, 0.000000000000000000, -2.259303855112193560E-12 ) ) ;
#23523=DIRECTION ( 'NONE',  ( 2.257144641404620116E-12, 2.777754792983395132E-24, 1.000000000000000000 ) ) ;
ENDSEC;
END-ISO-10303-21;
